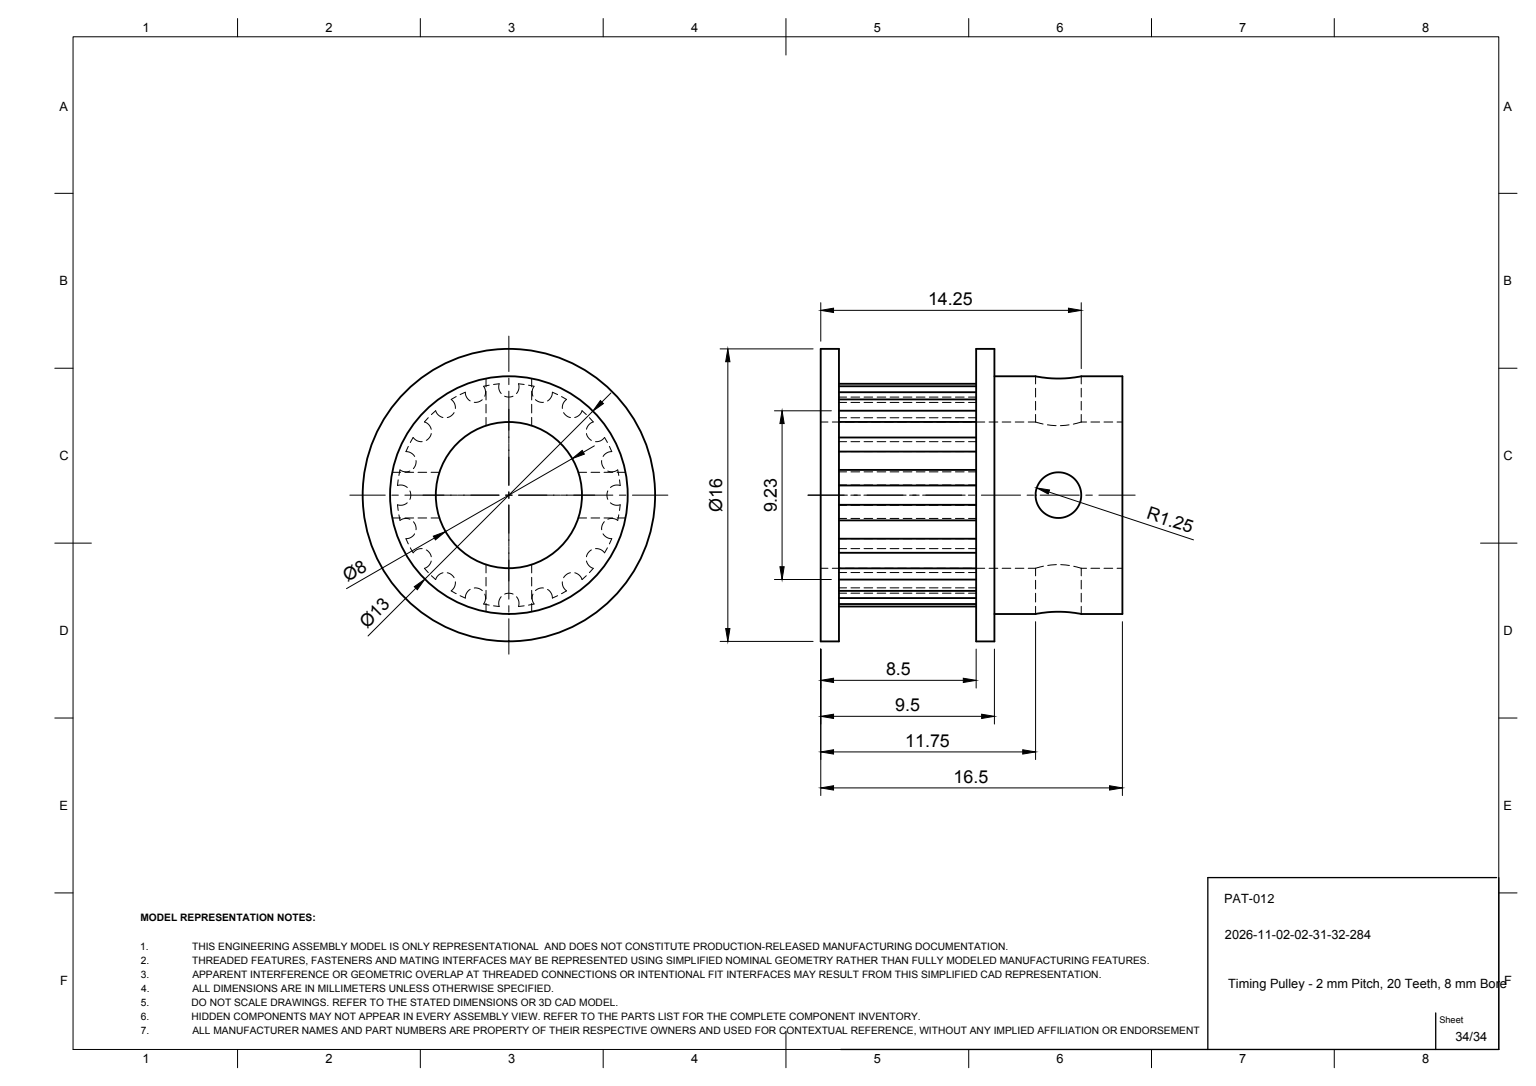
ISO-10303-21;
HEADER;
/* Generated by software containing ST-Developer
 * from STEP Tools, Inc. (www.steptools.com) 
 */

FILE_DESCRIPTION(
/* description */ ('Belt tensioner idler arm'),
/* implementation_level */ '2;1');

FILE_NAME(
/* name */ 'Timing Pulley - 2 mm Pitch, 20 Teeth, 8 mm Bore.step',
/* time_stamp */ '2026-10-28T03:22:15-07:00',
/* author */ (''),
/* organization */ (''),
/* preprocessor_version */ 'ST-DEVELOPER v20.2',
/* originating_system */ 'Autodesk Translation Framework v15.17.0.0',
/* authorisation */ '');

FILE_SCHEMA (('AUTOMOTIVE_DESIGN { 1 0 10303 214 3 1 1 }'));
ENDSEC;

DATA;
#10=MECHANICAL_DESIGN_GEOMETRIC_PRESENTATION_REPRESENTATION('',(#487),#12779);
#357=B_SPLINE_CURVE_WITH_KNOTS('',3,(#12023,#12024,#12025,#12026,#12027,
#12028,#12029,#12030,#12031,#12032),.UNSPECIFIED.,.F.,.F.,(4,2,2,2,4),(0.566550474129931,
0.613761886174531,0.66097329821913,0.708186965196186,0.755400632173242),
 .UNSPECIFIED.);
#358=B_SPLINE_CURVE_WITH_KNOTS('',3,(#12034,#12035,#12036,#12037,#12038,
#12039,#12040,#12041,#12042,#12043,#12044,#12045,#12046,#12047,#12048,#12049,
#12050,#12051),.UNSPECIFIED.,.F.,.F.,(4,2,2,2,2,2,2,2,4),(0.18885015804331,
0.23606157008791,0.283272982132509,0.330486649109565,0.377700316086621,
0.424913983063677,0.472127650040732,0.519339062085332,0.566550474129931),
 .UNSPECIFIED.);
#359=B_SPLINE_CURVE_WITH_KNOTS('',3,(#12052,#12053,#12054,#12055,#12056,
#12057,#12058,#12059,#12060,#12061),.UNSPECIFIED.,.F.,.F.,(4,2,2,2,4),(0.755400632173242,
0.802614299150298,0.849827966127353,0.897039378171953,0.944250790216552),
 .UNSPECIFIED.);
#360=B_SPLINE_CURVE_WITH_KNOTS('',3,(#12065,#12066,#12067,#12068,#12069,
#12070,#12071,#12072,#12073,#12074),.UNSPECIFIED.,.F.,.F.,(4,2,2,2,4),(0.189723673274825,
0.237146208024627,0.28456874277443,0.33200804466204,0.37944734654965),
 .UNSPECIFIED.);
#361=B_SPLINE_CURVE_WITH_KNOTS('',3,(#12076,#12077,#12078,#12079,#12080,
#12081,#12082,#12083,#12084,#12085),.UNSPECIFIED.,.F.,.F.,(4,2,2,2,4),(0.,
0.0474393018876097,0.0948786037752193,0.142301138525022,0.189723673274825),
 .UNSPECIFIED.);
#362=B_SPLINE_CURVE_WITH_KNOTS('',3,(#12087,#12088,#12089,#12090,#12091,
#12092,#12093,#12094,#12095,#12096),.UNSPECIFIED.,.F.,.F.,(4,2,2,2,4),(0.569171019824474,
0.616593554574277,0.66401608932408,0.711455391211689,0.758894693099299),
 .UNSPECIFIED.);
#363=B_SPLINE_CURVE_WITH_KNOTS('',3,(#12097,#12098,#12099,#12100,#12101,
#12102,#12103,#12104,#12105,#12106),.UNSPECIFIED.,.F.,.F.,(4,2,2,2,4),(0.37944734654965,
0.426886648437259,0.474325950324869,0.521748485074671,0.569171019824474),
 .UNSPECIFIED.);
#364=B_SPLINE_CURVE_WITH_KNOTS('',3,(#12110,#12111,#12112,#12113,#12114,
#12115,#12116,#12117,#12118,#12119,#12120,#12121,#12122,#12123,#12124,#12125,
#12126,#12127),.UNSPECIFIED.,.F.,.F.,(4,2,2,2,2,2,2,2,4),(0.,0.0474393018876097,
0.0948786037752194,0.142301138525022,0.189723673274825,0.237146208024628,
0.28456874277443,0.33200804466204,0.37944734654965),.UNSPECIFIED.);
#365=B_SPLINE_CURVE_WITH_KNOTS('',3,(#12128,#12129,#12130,#12131,#12132,
#12133,#12134,#12135,#12136,#12137,#12138,#12139,#12140,#12141,#12142,#12143,
#12144,#12145),.UNSPECIFIED.,.F.,.F.,(4,2,2,2,2,2,2,2,4),(0.37944734654965,
0.426886648437259,0.474325950324869,0.521748485074672,0.569171019824474,
0.616593554574277,0.66401608932408,0.711455391211689,0.758894693099299),
 .UNSPECIFIED.);
#366=B_SPLINE_CURVE_WITH_KNOTS('',3,(#12149,#12150,#12151,#12152,#12153,
#12154,#12155,#12156,#12157,#12158),.UNSPECIFIED.,.F.,.F.,(4,2,2,2,4),(0.566550474129931,
0.613761886174531,0.66097329821913,0.708186965196186,0.755400632173242),
 .UNSPECIFIED.);
#367=B_SPLINE_CURVE_WITH_KNOTS('',3,(#12160,#12161,#12162,#12163,#12164,
#12165,#12166,#12167,#12168,#12169,#12170,#12171,#12172,#12173,#12174,#12175,
#12176,#12177),.UNSPECIFIED.,.F.,.F.,(4,2,2,2,2,2,2,2,4),(0.188850158043311,
0.23606157008791,0.283272982132509,0.330486649109565,0.377700316086621,
0.424913983063677,0.472127650040733,0.519339062085332,0.566550474129931),
 .UNSPECIFIED.);
#368=B_SPLINE_CURVE_WITH_KNOTS('',3,(#12178,#12179,#12180,#12181,#12182,
#12183,#12184,#12185,#12186,#12187),.UNSPECIFIED.,.F.,.F.,(4,2,2,2,4),(0.755400632173242,
0.802614299150298,0.849827966127354,0.897039378171953,0.944250790216552),
 .UNSPECIFIED.);
#369=B_SPLINE_CURVE_WITH_KNOTS('',3,(#12197,#12198,#12199,#12200,#12201,
#12202,#12203,#12204,#12205,#12206,#12207,#12208,#12209,#12210,#12211,#12212,
#12213,#12214),.UNSPECIFIED.,.F.,.F.,(4,2,2,2,2,2,2,2,4),(0.18885015804331,
0.23606157008791,0.283272982132509,0.330486649109565,0.377700316086621,
0.424913983063677,0.472127650040732,0.519339062085332,0.566550474129931),
 .UNSPECIFIED.);
#370=B_SPLINE_CURVE_WITH_KNOTS('',3,(#12216,#12217,#12218,#12219,#12220,
#12221,#12222,#12223,#12224,#12225),.UNSPECIFIED.,.F.,.F.,(4,2,2,2,4),(0.566550474129931,
0.613761886174531,0.66097329821913,0.708186965196186,0.755400632173242),
 .UNSPECIFIED.);
#371=B_SPLINE_CURVE_WITH_KNOTS('',3,(#12226,#12227,#12228,#12229,#12230,
#12231,#12232,#12233,#12234,#12235),.UNSPECIFIED.,.F.,.F.,(4,2,2,2,4),(0.755400632173242,
0.802614299150298,0.849827966127353,0.897039378171953,0.944250790216552),
 .UNSPECIFIED.);
#372=B_SPLINE_CURVE_WITH_KNOTS('',3,(#12238,#12239,#12240,#12241,#12242,
#12243,#12244,#12245,#12246,#12247,#12248,#12249,#12250,#12251,#12252,#12253,
#12254,#12255),.UNSPECIFIED.,.F.,.F.,(4,2,2,2,2,2,2,2,4),(0.188850158043311,
0.23606157008791,0.283272982132509,0.330486649109565,0.377700316086621,
0.424913983063677,0.472127650040733,0.519339062085332,0.566550474129932),
 .UNSPECIFIED.);
#373=B_SPLINE_CURVE_WITH_KNOTS('',3,(#12257,#12258,#12259,#12260,#12261,
#12262,#12263,#12264,#12265,#12266),.UNSPECIFIED.,.F.,.F.,(4,2,2,2,4),(0.566550474129932,
0.613761886174531,0.66097329821913,0.708186965196186,0.755400632173242),
 .UNSPECIFIED.);
#374=B_SPLINE_CURVE_WITH_KNOTS('',3,(#12267,#12268,#12269,#12270,#12271,
#12272,#12273,#12274,#12275,#12276),.UNSPECIFIED.,.F.,.F.,(4,2,2,2,4),(0.755400632173242,
0.802614299150298,0.849827966127354,0.897039378171953,0.944250790216552),
 .UNSPECIFIED.);
#375=B_SPLINE_CURVE_WITH_KNOTS('',3,(#12281,#12282,#12283,#12284,#12285,
#12286,#12287,#12288,#12289,#12290,#12291,#12292,#12293,#12294,#12295,#12296,
#12297,#12298),.UNSPECIFIED.,.F.,.F.,(4,2,2,2,2,2,2,2,4),(0.,0.0474393018876097,
0.0948786037752193,0.142301138525022,0.189723673274825,0.237146208024627,
0.28456874277443,0.33200804466204,0.37944734654965),.UNSPECIFIED.);
#376=B_SPLINE_CURVE_WITH_KNOTS('',3,(#12299,#12300,#12301,#12302,#12303,
#12304,#12305,#12306,#12307,#12308,#12309,#12310,#12311,#12312,#12313,#12314,
#12315,#12316),.UNSPECIFIED.,.F.,.F.,(4,2,2,2,2,2,2,2,4),(0.37944734654965,
0.426886648437259,0.474325950324869,0.521748485074672,0.569171019824474,
0.616593554574277,0.66401608932408,0.711455391211689,0.758894693099299),
 .UNSPECIFIED.);
#377=B_SPLINE_CURVE_WITH_KNOTS('',3,(#12320,#12321,#12322,#12323,#12324,
#12325,#12326,#12327,#12328,#12329,#12330,#12331,#12332,#12333,#12334,#12335,
#12336,#12337),.UNSPECIFIED.,.F.,.F.,(4,2,2,2,2,2,2,2,4),(0.,0.0474393018876097,
0.0948786037752194,0.142301138525022,0.189723673274825,0.237146208024627,
0.28456874277443,0.33200804466204,0.37944734654965),.UNSPECIFIED.);
#378=B_SPLINE_CURVE_WITH_KNOTS('',3,(#12338,#12339,#12340,#12341,#12342,
#12343,#12344,#12345,#12346,#12347,#12348,#12349,#12350,#12351,#12352,#12353,
#12354,#12355),.UNSPECIFIED.,.F.,.F.,(4,2,2,2,2,2,2,2,4),(0.37944734654965,
0.426886648437259,0.474325950324869,0.521748485074672,0.569171019824474,
0.616593554574277,0.66401608932408,0.711455391211689,0.758894693099299),
 .UNSPECIFIED.);
#411=SHAPE_REPRESENTATION_RELATIONSHIP('SRR','None',#12960,#445);
#445=ADVANCED_BREP_SHAPE_REPRESENTATION('',(#526),#12777);
#487=STYLED_ITEM('',(#13198),#526);
#526=MANIFOLD_SOLID_BREP('Body1',#6224);
#651=FACE_BOUND('',#1629,.T.);
#652=FACE_BOUND('',#1630,.T.);
#653=FACE_BOUND('',#1631,.T.);
#654=FACE_BOUND('',#1635,.T.);
#655=FACE_BOUND('',#1636,.T.);
#656=FACE_BOUND('',#1637,.T.);
#657=FACE_BOUND('',#1639,.T.);
#658=FACE_BOUND('',#1641,.T.);
#659=FACE_BOUND('',#1644,.T.);
#660=FACE_BOUND('',#1646,.T.);
#661=FACE_BOUND('',#1649,.T.);
#821=PLANE('',#7265);
#822=PLANE('',#7266);
#823=PLANE('',#7310);
#824=PLANE('',#7311);
#825=PLANE('',#7355);
#1135=FACE_OUTER_BOUND('',#1626,.T.);
#1136=FACE_OUTER_BOUND('',#1627,.T.);
#1137=FACE_OUTER_BOUND('',#1628,.T.);
#1138=FACE_OUTER_BOUND('',#1632,.T.);
#1139=FACE_OUTER_BOUND('',#1633,.T.);
#1140=FACE_OUTER_BOUND('',#1634,.T.);
#1141=FACE_OUTER_BOUND('',#1638,.T.);
#1142=FACE_OUTER_BOUND('',#1640,.T.);
#1143=FACE_OUTER_BOUND('',#1642,.T.);
#1144=FACE_OUTER_BOUND('',#1643,.T.);
#1145=FACE_OUTER_BOUND('',#1645,.T.);
#1146=FACE_OUTER_BOUND('',#1647,.T.);
#1147=FACE_OUTER_BOUND('',#1648,.T.);
#1148=FACE_OUTER_BOUND('',#1650,.T.);
#1149=FACE_OUTER_BOUND('',#1651,.T.);
#1150=FACE_OUTER_BOUND('',#1652,.T.);
#1151=FACE_OUTER_BOUND('',#1653,.T.);
#1152=FACE_OUTER_BOUND('',#1654,.T.);
#1153=FACE_OUTER_BOUND('',#1655,.T.);
#1154=FACE_OUTER_BOUND('',#1656,.T.);
#1155=FACE_OUTER_BOUND('',#1657,.T.);
#1156=FACE_OUTER_BOUND('',#1658,.T.);
#1157=FACE_OUTER_BOUND('',#1659,.T.);
#1158=FACE_OUTER_BOUND('',#1660,.T.);
#1159=FACE_OUTER_BOUND('',#1661,.T.);
#1160=FACE_OUTER_BOUND('',#1662,.T.);
#1161=FACE_OUTER_BOUND('',#1663,.T.);
#1162=FACE_OUTER_BOUND('',#1664,.T.);
#1163=FACE_OUTER_BOUND('',#1665,.T.);
#1164=FACE_OUTER_BOUND('',#1666,.T.);
#1165=FACE_OUTER_BOUND('',#1667,.T.);
#1166=FACE_OUTER_BOUND('',#1668,.T.);
#1167=FACE_OUTER_BOUND('',#1669,.T.);
#1168=FACE_OUTER_BOUND('',#1670,.T.);
#1169=FACE_OUTER_BOUND('',#1671,.T.);
#1170=FACE_OUTER_BOUND('',#1672,.T.);
#1171=FACE_OUTER_BOUND('',#1673,.T.);
#1172=FACE_OUTER_BOUND('',#1674,.T.);
#1173=FACE_OUTER_BOUND('',#1675,.T.);
#1174=FACE_OUTER_BOUND('',#1676,.T.);
#1175=FACE_OUTER_BOUND('',#1677,.T.);
#1176=FACE_OUTER_BOUND('',#1678,.T.);
#1177=FACE_OUTER_BOUND('',#1679,.T.);
#1178=FACE_OUTER_BOUND('',#1680,.T.);
#1179=FACE_OUTER_BOUND('',#1681,.T.);
#1180=FACE_OUTER_BOUND('',#1682,.T.);
#1181=FACE_OUTER_BOUND('',#1683,.T.);
#1182=FACE_OUTER_BOUND('',#1684,.T.);
#1183=FACE_OUTER_BOUND('',#1685,.T.);
#1184=FACE_OUTER_BOUND('',#1686,.T.);
#1185=FACE_OUTER_BOUND('',#1687,.T.);
#1186=FACE_OUTER_BOUND('',#1688,.T.);
#1187=FACE_OUTER_BOUND('',#1689,.T.);
#1626=EDGE_LOOP('',(#5282,#5283,#5284,#5285,#5286,#5287,#5288,#5289,#5290));
#1627=EDGE_LOOP('',(#5291,#5292,#5293,#5294,#5295,#5296,#5297));
#1628=EDGE_LOOP('',(#5298,#5299,#5300,#5301,#5302,#5303,#5304,#5305,#5306));
#1629=EDGE_LOOP('',(#5307,#5308,#5309));
#1630=EDGE_LOOP('',(#5310,#5311,#5312));
#1631=EDGE_LOOP('',(#5313,#5314,#5315));
#1632=EDGE_LOOP('',(#5316,#5317,#5318,#5319,#5320,#5321,#5322));
#1633=EDGE_LOOP('',(#5323,#5324,#5325,#5326,#5327,#5328,#5329));
#1634=EDGE_LOOP('',(#5330,#5331,#5332,#5333,#5334,#5335,#5336,#5337,#5338,
#5339));
#1635=EDGE_LOOP('',(#5340,#5341));
#1636=EDGE_LOOP('',(#5342,#5343));
#1637=EDGE_LOOP('',(#5344,#5345));
#1638=EDGE_LOOP('',(#5346));
#1639=EDGE_LOOP('',(#5347));
#1640=EDGE_LOOP('',(#5348));
#1641=EDGE_LOOP('',(#5349,#5350,#5351,#5352,#5353,#5354,#5355,#5356,#5357,
#5358,#5359,#5360,#5361,#5362,#5363,#5364,#5365,#5366,#5367,#5368,#5369,
#5370,#5371,#5372,#5373,#5374,#5375,#5376,#5377,#5378,#5379,#5380,#5381,
#5382,#5383,#5384,#5385,#5386,#5387,#5388));
#1642=EDGE_LOOP('',(#5389,#5390,#5391,#5392));
#1643=EDGE_LOOP('',(#5393));
#1644=EDGE_LOOP('',(#5394));
#1645=EDGE_LOOP('',(#5395));
#1646=EDGE_LOOP('',(#5396,#5397,#5398,#5399,#5400,#5401,#5402,#5403,#5404,
#5405,#5406,#5407,#5408,#5409,#5410,#5411,#5412,#5413,#5414,#5415,#5416,
#5417,#5418,#5419,#5420,#5421,#5422,#5423,#5424,#5425,#5426,#5427,#5428,
#5429,#5430,#5431,#5432,#5433,#5434,#5435));
#1647=EDGE_LOOP('',(#5436,#5437,#5438,#5439));
#1648=EDGE_LOOP('',(#5440));
#1649=EDGE_LOOP('',(#5441));
#1650=EDGE_LOOP('',(#5442,#5443,#5444,#5445));
#1651=EDGE_LOOP('',(#5446,#5447,#5448,#5449));
#1652=EDGE_LOOP('',(#5450,#5451,#5452,#5453));
#1653=EDGE_LOOP('',(#5454,#5455,#5456,#5457));
#1654=EDGE_LOOP('',(#5458,#5459,#5460,#5461));
#1655=EDGE_LOOP('',(#5462,#5463,#5464,#5465));
#1656=EDGE_LOOP('',(#5466,#5467,#5468,#5469));
#1657=EDGE_LOOP('',(#5470,#5471,#5472,#5473));
#1658=EDGE_LOOP('',(#5474,#5475,#5476,#5477));
#1659=EDGE_LOOP('',(#5478,#5479,#5480,#5481));
#1660=EDGE_LOOP('',(#5482,#5483,#5484,#5485));
#1661=EDGE_LOOP('',(#5486,#5487,#5488,#5489));
#1662=EDGE_LOOP('',(#5490,#5491,#5492,#5493));
#1663=EDGE_LOOP('',(#5494,#5495,#5496,#5497));
#1664=EDGE_LOOP('',(#5498,#5499,#5500,#5501));
#1665=EDGE_LOOP('',(#5502,#5503,#5504,#5505));
#1666=EDGE_LOOP('',(#5506,#5507,#5508,#5509));
#1667=EDGE_LOOP('',(#5510,#5511,#5512,#5513));
#1668=EDGE_LOOP('',(#5514,#5515,#5516,#5517));
#1669=EDGE_LOOP('',(#5518,#5519,#5520,#5521));
#1670=EDGE_LOOP('',(#5522,#5523,#5524,#5525));
#1671=EDGE_LOOP('',(#5526,#5527,#5528,#5529));
#1672=EDGE_LOOP('',(#5530,#5531,#5532,#5533));
#1673=EDGE_LOOP('',(#5534,#5535,#5536,#5537));
#1674=EDGE_LOOP('',(#5538,#5539,#5540,#5541));
#1675=EDGE_LOOP('',(#5542,#5543,#5544,#5545));
#1676=EDGE_LOOP('',(#5546,#5547,#5548,#5549));
#1677=EDGE_LOOP('',(#5550,#5551,#5552,#5553));
#1678=EDGE_LOOP('',(#5554,#5555,#5556,#5557));
#1679=EDGE_LOOP('',(#5558,#5559,#5560,#5561));
#1680=EDGE_LOOP('',(#5562,#5563,#5564,#5565));
#1681=EDGE_LOOP('',(#5566,#5567,#5568,#5569));
#1682=EDGE_LOOP('',(#5570,#5571,#5572,#5573));
#1683=EDGE_LOOP('',(#5574,#5575,#5576,#5577));
#1684=EDGE_LOOP('',(#5578,#5579,#5580,#5581));
#1685=EDGE_LOOP('',(#5582,#5583,#5584,#5585));
#1686=EDGE_LOOP('',(#5586,#5587,#5588,#5589));
#1687=EDGE_LOOP('',(#5590,#5591,#5592,#5593));
#1688=EDGE_LOOP('',(#5594,#5595,#5596,#5597));
#1689=EDGE_LOOP('',(#5598,#5599,#5600,#5601));
#1983=LINE('',#12063,#2332);
#1984=LINE('',#12147,#2333);
#1985=LINE('',#12191,#2334);
#1986=LINE('',#12193,#2335);
#1987=LINE('',#12279,#2336);
#1988=LINE('',#12356,#2337);
#1989=LINE('',#12360,#2338);
#1990=LINE('',#12362,#2339);
#1991=LINE('',#12451,#2340);
#1992=LINE('',#12539,#2341);
#1993=LINE('',#12542,#2342);
#1994=LINE('',#12543,#2343);
#1995=LINE('',#12545,#2344);
#1996=LINE('',#12547,#2345);
#1997=LINE('',#12549,#2346);
#1998=LINE('',#12551,#2347);
#1999=LINE('',#12553,#2348);
#2000=LINE('',#12555,#2349);
#2001=LINE('',#12557,#2350);
#2002=LINE('',#12559,#2351);
#2003=LINE('',#12561,#2352);
#2004=LINE('',#12563,#2353);
#2005=LINE('',#12565,#2354);
#2006=LINE('',#12567,#2355);
#2007=LINE('',#12569,#2356);
#2008=LINE('',#12571,#2357);
#2009=LINE('',#12573,#2358);
#2010=LINE('',#12575,#2359);
#2011=LINE('',#12577,#2360);
#2012=LINE('',#12579,#2361);
#2013=LINE('',#12581,#2362);
#2014=LINE('',#12583,#2363);
#2015=LINE('',#12585,#2364);
#2016=LINE('',#12587,#2365);
#2017=LINE('',#12589,#2366);
#2018=LINE('',#12591,#2367);
#2019=LINE('',#12593,#2368);
#2020=LINE('',#12595,#2369);
#2021=LINE('',#12597,#2370);
#2022=LINE('',#12599,#2371);
#2023=LINE('',#12601,#2372);
#2024=LINE('',#12603,#2373);
#2025=LINE('',#12605,#2374);
#2026=LINE('',#12607,#2375);
#2027=LINE('',#12609,#2376);
#2028=LINE('',#12611,#2377);
#2029=LINE('',#12613,#2378);
#2030=LINE('',#12615,#2379);
#2031=LINE('',#12617,#2380);
#2032=LINE('',#12619,#2381);
#2332=VECTOR('',#9017,0.125);
#2333=VECTOR('',#9020,0.125);
#2334=VECTOR('',#9025,0.65);
#2335=VECTOR('',#9026,0.65);
#2336=VECTOR('',#9031,0.125);
#2337=VECTOR('',#9034,0.125);
#2338=VECTOR('',#9039,0.4);
#2339=VECTOR('',#9040,0.4);
#2340=VECTOR('',#9133,0.8);
#2341=VECTOR('',#9224,0.8);
#2342=VECTOR('',#9229,1.);
#2343=VECTOR('',#9230,1.);
#2344=VECTOR('',#9233,1.);
#2345=VECTOR('',#9236,1.);
#2346=VECTOR('',#9239,1.);
#2347=VECTOR('',#9242,1.);
#2348=VECTOR('',#9245,1.);
#2349=VECTOR('',#9248,1.);
#2350=VECTOR('',#9251,1.);
#2351=VECTOR('',#9254,1.);
#2352=VECTOR('',#9257,1.);
#2353=VECTOR('',#9260,1.);
#2354=VECTOR('',#9263,1.);
#2355=VECTOR('',#9266,1.);
#2356=VECTOR('',#9269,1.);
#2357=VECTOR('',#9272,1.);
#2358=VECTOR('',#9275,1.);
#2359=VECTOR('',#9278,1.);
#2360=VECTOR('',#9281,1.);
#2361=VECTOR('',#9284,1.);
#2362=VECTOR('',#9287,1.);
#2363=VECTOR('',#9290,1.);
#2364=VECTOR('',#9293,1.);
#2365=VECTOR('',#9296,1.);
#2366=VECTOR('',#9299,1.);
#2367=VECTOR('',#9302,1.);
#2368=VECTOR('',#9305,1.);
#2369=VECTOR('',#9308,1.);
#2370=VECTOR('',#9311,1.);
#2371=VECTOR('',#9314,1.);
#2372=VECTOR('',#9317,1.);
#2373=VECTOR('',#9320,1.);
#2374=VECTOR('',#9323,1.);
#2375=VECTOR('',#9326,1.);
#2376=VECTOR('',#9329,1.);
#2377=VECTOR('',#9332,1.);
#2378=VECTOR('',#9335,1.);
#2379=VECTOR('',#9338,1.);
#2380=VECTOR('',#9341,1.);
#2381=VECTOR('',#9344,1.);
#2674=CIRCLE('',#7258,0.65);
#2675=CIRCLE('',#7259,0.65);
#2676=CIRCLE('',#7263,0.4);
#2677=CIRCLE('',#7264,0.4);
#2678=CIRCLE('',#7267,0.8);
#2679=CIRCLE('',#7268,0.0555);
#2680=CIRCLE('',#7269,0.611219772367581);
#2681=CIRCLE('',#7270,0.0555);
#2682=CIRCLE('',#7271,0.611219772367581);
#2683=CIRCLE('',#7272,0.0555);
#2684=CIRCLE('',#7273,0.611219772367581);
#2685=CIRCLE('',#7274,0.0555);
#2686=CIRCLE('',#7275,0.611219772367581);
#2687=CIRCLE('',#7276,0.0555);
#2688=CIRCLE('',#7277,0.611219772367581);
#2689=CIRCLE('',#7278,0.0555);
#2690=CIRCLE('',#7279,0.611219772367581);
#2691=CIRCLE('',#7280,0.0555);
#2692=CIRCLE('',#7281,0.611219772367581);
#2693=CIRCLE('',#7282,0.0555);
#2694=CIRCLE('',#7283,0.611219772367581);
#2695=CIRCLE('',#7284,0.0555);
#2696=CIRCLE('',#7285,0.611219772367581);
#2697=CIRCLE('',#7286,0.0555);
#2698=CIRCLE('',#7287,0.611219772367581);
#2699=CIRCLE('',#7288,0.0555);
#2700=CIRCLE('',#7289,0.611219772367581);
#2701=CIRCLE('',#7290,0.0555);
#2702=CIRCLE('',#7291,0.611219772367581);
#2703=CIRCLE('',#7292,0.0555);
#2704=CIRCLE('',#7293,0.611219772367581);
#2705=CIRCLE('',#7294,0.0555);
#2706=CIRCLE('',#7295,0.611219772367581);
#2707=CIRCLE('',#7296,0.0555);
#2708=CIRCLE('',#7297,0.611219772367581);
#2709=CIRCLE('',#7298,0.0555);
#2710=CIRCLE('',#7299,0.611219772367581);
#2711=CIRCLE('',#7300,0.0555);
#2712=CIRCLE('',#7301,0.611219772367581);
#2713=CIRCLE('',#7302,0.0555);
#2714=CIRCLE('',#7303,0.611219772367581);
#2715=CIRCLE('',#7304,0.0555);
#2716=CIRCLE('',#7305,0.611219772367581);
#2717=CIRCLE('',#7306,0.0555);
#2718=CIRCLE('',#7307,0.611219772367581);
#2719=CIRCLE('',#7309,0.8);
#2720=CIRCLE('',#7312,0.8);
#2721=CIRCLE('',#7313,0.0555);
#2722=CIRCLE('',#7314,0.611219772367581);
#2723=CIRCLE('',#7315,0.0555);
#2724=CIRCLE('',#7316,0.611219772367581);
#2725=CIRCLE('',#7317,0.0555);
#2726=CIRCLE('',#7318,0.611219772367581);
#2727=CIRCLE('',#7319,0.0555);
#2728=CIRCLE('',#7320,0.611219772367581);
#2729=CIRCLE('',#7321,0.0555);
#2730=CIRCLE('',#7322,0.611219772367581);
#2731=CIRCLE('',#7323,0.0555);
#2732=CIRCLE('',#7324,0.611219772367581);
#2733=CIRCLE('',#7325,0.0555);
#2734=CIRCLE('',#7326,0.611219772367581);
#2735=CIRCLE('',#7327,0.0555);
#2736=CIRCLE('',#7328,0.611219772367581);
#2737=CIRCLE('',#7329,0.0555);
#2738=CIRCLE('',#7330,0.611219772367581);
#2739=CIRCLE('',#7331,0.0555);
#2740=CIRCLE('',#7332,0.611219772367581);
#2741=CIRCLE('',#7333,0.0555);
#2742=CIRCLE('',#7334,0.611219772367581);
#2743=CIRCLE('',#7335,0.0555);
#2744=CIRCLE('',#7336,0.611219772367581);
#2745=CIRCLE('',#7337,0.0555);
#2746=CIRCLE('',#7338,0.611219772367581);
#2747=CIRCLE('',#7339,0.0555);
#2748=CIRCLE('',#7340,0.611219772367581);
#2749=CIRCLE('',#7341,0.0555);
#2750=CIRCLE('',#7342,0.611219772367581);
#2751=CIRCLE('',#7343,0.0555);
#2752=CIRCLE('',#7344,0.611219772367581);
#2753=CIRCLE('',#7345,0.0555);
#2754=CIRCLE('',#7346,0.611219772367581);
#2755=CIRCLE('',#7347,0.0555);
#2756=CIRCLE('',#7348,0.611219772367581);
#2757=CIRCLE('',#7349,0.0555);
#2758=CIRCLE('',#7350,0.611219772367581);
#2759=CIRCLE('',#7351,0.0555);
#2760=CIRCLE('',#7352,0.611219772367581);
#2761=CIRCLE('',#7354,0.8);
#3169=VERTEX_POINT('',#12021);
#3170=VERTEX_POINT('',#12022);
#3171=VERTEX_POINT('',#12033);
#3172=VERTEX_POINT('',#12062);
#3173=VERTEX_POINT('',#12064);
#3174=VERTEX_POINT('',#12075);
#3175=VERTEX_POINT('',#12086);
#3176=VERTEX_POINT('',#12108);
#3177=VERTEX_POINT('',#12109);
#3178=VERTEX_POINT('',#12146);
#3179=VERTEX_POINT('',#12148);
#3180=VERTEX_POINT('',#12159);
#3181=VERTEX_POINT('',#12189);
#3182=VERTEX_POINT('',#12192);
#3183=VERTEX_POINT('',#12195);
#3184=VERTEX_POINT('',#12196);
#3185=VERTEX_POINT('',#12215);
#3186=VERTEX_POINT('',#12236);
#3187=VERTEX_POINT('',#12237);
#3188=VERTEX_POINT('',#12256);
#3189=VERTEX_POINT('',#12278);
#3190=VERTEX_POINT('',#12280);
#3191=VERTEX_POINT('',#12318);
#3192=VERTEX_POINT('',#12319);
#3193=VERTEX_POINT('',#12358);
#3194=VERTEX_POINT('',#12361);
#3195=VERTEX_POINT('',#12366);
#3196=VERTEX_POINT('',#12368);
#3197=VERTEX_POINT('',#12369);
#3198=VERTEX_POINT('',#12371);
#3199=VERTEX_POINT('',#12373);
#3200=VERTEX_POINT('',#12375);
#3201=VERTEX_POINT('',#12377);
#3202=VERTEX_POINT('',#12379);
#3203=VERTEX_POINT('',#12381);
#3204=VERTEX_POINT('',#12383);
#3205=VERTEX_POINT('',#12385);
#3206=VERTEX_POINT('',#12387);
#3207=VERTEX_POINT('',#12389);
#3208=VERTEX_POINT('',#12391);
#3209=VERTEX_POINT('',#12393);
#3210=VERTEX_POINT('',#12395);
#3211=VERTEX_POINT('',#12397);
#3212=VERTEX_POINT('',#12399);
#3213=VERTEX_POINT('',#12401);
#3214=VERTEX_POINT('',#12403);
#3215=VERTEX_POINT('',#12405);
#3216=VERTEX_POINT('',#12407);
#3217=VERTEX_POINT('',#12409);
#3218=VERTEX_POINT('',#12411);
#3219=VERTEX_POINT('',#12413);
#3220=VERTEX_POINT('',#12415);
#3221=VERTEX_POINT('',#12417);
#3222=VERTEX_POINT('',#12419);
#3223=VERTEX_POINT('',#12421);
#3224=VERTEX_POINT('',#12423);
#3225=VERTEX_POINT('',#12425);
#3226=VERTEX_POINT('',#12427);
#3227=VERTEX_POINT('',#12429);
#3228=VERTEX_POINT('',#12431);
#3229=VERTEX_POINT('',#12433);
#3230=VERTEX_POINT('',#12435);
#3231=VERTEX_POINT('',#12437);
#3232=VERTEX_POINT('',#12439);
#3233=VERTEX_POINT('',#12441);
#3234=VERTEX_POINT('',#12443);
#3235=VERTEX_POINT('',#12445);
#3236=VERTEX_POINT('',#12449);
#3237=VERTEX_POINT('',#12454);
#3238=VERTEX_POINT('',#12456);
#3239=VERTEX_POINT('',#12457);
#3240=VERTEX_POINT('',#12459);
#3241=VERTEX_POINT('',#12461);
#3242=VERTEX_POINT('',#12463);
#3243=VERTEX_POINT('',#12465);
#3244=VERTEX_POINT('',#12467);
#3245=VERTEX_POINT('',#12469);
#3246=VERTEX_POINT('',#12471);
#3247=VERTEX_POINT('',#12473);
#3248=VERTEX_POINT('',#12475);
#3249=VERTEX_POINT('',#12477);
#3250=VERTEX_POINT('',#12479);
#3251=VERTEX_POINT('',#12481);
#3252=VERTEX_POINT('',#12483);
#3253=VERTEX_POINT('',#12485);
#3254=VERTEX_POINT('',#12487);
#3255=VERTEX_POINT('',#12489);
#3256=VERTEX_POINT('',#12491);
#3257=VERTEX_POINT('',#12493);
#3258=VERTEX_POINT('',#12495);
#3259=VERTEX_POINT('',#12497);
#3260=VERTEX_POINT('',#12499);
#3261=VERTEX_POINT('',#12501);
#3262=VERTEX_POINT('',#12503);
#3263=VERTEX_POINT('',#12505);
#3264=VERTEX_POINT('',#12507);
#3265=VERTEX_POINT('',#12509);
#3266=VERTEX_POINT('',#12511);
#3267=VERTEX_POINT('',#12513);
#3268=VERTEX_POINT('',#12515);
#3269=VERTEX_POINT('',#12517);
#3270=VERTEX_POINT('',#12519);
#3271=VERTEX_POINT('',#12521);
#3272=VERTEX_POINT('',#12523);
#3273=VERTEX_POINT('',#12525);
#3274=VERTEX_POINT('',#12527);
#3275=VERTEX_POINT('',#12529);
#3276=VERTEX_POINT('',#12531);
#3277=VERTEX_POINT('',#12533);
#3278=VERTEX_POINT('',#12537);
#3896=EDGE_CURVE('',#3169,#3170,#357,.T.);
#3897=EDGE_CURVE('',#3171,#3169,#358,.T.);
#3898=EDGE_CURVE('',#3170,#3171,#359,.T.);
#3899=EDGE_CURVE('',#3170,#3172,#1983,.T.);
#3900=EDGE_CURVE('',#3173,#3172,#360,.T.);
#3901=EDGE_CURVE('',#3174,#3173,#361,.T.);
#3902=EDGE_CURVE('',#3175,#3174,#362,.T.);
#3903=EDGE_CURVE('',#3172,#3175,#363,.T.);
#3904=EDGE_CURVE('',#3176,#3177,#364,.T.);
#3905=EDGE_CURVE('',#3177,#3176,#365,.T.);
#3906=EDGE_CURVE('',#3177,#3178,#1984,.T.);
#3907=EDGE_CURVE('',#3179,#3178,#366,.T.);
#3908=EDGE_CURVE('',#3180,#3179,#367,.T.);
#3909=EDGE_CURVE('',#3178,#3180,#368,.T.);
#3910=EDGE_CURVE('',#3181,#3181,#2674,.T.);
#3911=EDGE_CURVE('',#3181,#3171,#1985,.T.);
#3912=EDGE_CURVE('',#3169,#3182,#1986,.T.);
#3913=EDGE_CURVE('',#3182,#3182,#2675,.T.);
#3914=EDGE_CURVE('',#3183,#3184,#369,.T.);
#3915=EDGE_CURVE('',#3184,#3185,#370,.T.);
#3916=EDGE_CURVE('',#3185,#3183,#371,.T.);
#3917=EDGE_CURVE('',#3186,#3187,#372,.T.);
#3918=EDGE_CURVE('',#3187,#3188,#373,.T.);
#3919=EDGE_CURVE('',#3188,#3186,#374,.T.);
#3920=EDGE_CURVE('',#3185,#3189,#1987,.T.);
#3921=EDGE_CURVE('',#3190,#3189,#375,.T.);
#3922=EDGE_CURVE('',#3189,#3190,#376,.T.);
#3923=EDGE_CURVE('',#3191,#3192,#377,.T.);
#3924=EDGE_CURVE('',#3192,#3191,#378,.T.);
#3925=EDGE_CURVE('',#3192,#3188,#1988,.T.);
#3926=EDGE_CURVE('',#3193,#3193,#2676,.T.);
#3927=EDGE_CURVE('',#3193,#3173,#1989,.T.);
#3928=EDGE_CURVE('',#3175,#3194,#1990,.T.);
#3929=EDGE_CURVE('',#3194,#3194,#2677,.T.);
#3930=EDGE_CURVE('',#3195,#3195,#2678,.T.);
#3931=EDGE_CURVE('',#3196,#3197,#2679,.T.);
#3932=EDGE_CURVE('',#3198,#3197,#2680,.T.);
#3933=EDGE_CURVE('',#3198,#3199,#2681,.T.);
#3934=EDGE_CURVE('',#3200,#3199,#2682,.T.);
#3935=EDGE_CURVE('',#3200,#3201,#2683,.T.);
#3936=EDGE_CURVE('',#3202,#3201,#2684,.T.);
#3937=EDGE_CURVE('',#3202,#3203,#2685,.T.);
#3938=EDGE_CURVE('',#3204,#3203,#2686,.T.);
#3939=EDGE_CURVE('',#3204,#3205,#2687,.T.);
#3940=EDGE_CURVE('',#3206,#3205,#2688,.T.);
#3941=EDGE_CURVE('',#3206,#3207,#2689,.T.);
#3942=EDGE_CURVE('',#3208,#3207,#2690,.T.);
#3943=EDGE_CURVE('',#3208,#3209,#2691,.T.);
#3944=EDGE_CURVE('',#3210,#3209,#2692,.T.);
#3945=EDGE_CURVE('',#3210,#3211,#2693,.T.);
#3946=EDGE_CURVE('',#3212,#3211,#2694,.T.);
#3947=EDGE_CURVE('',#3212,#3213,#2695,.T.);
#3948=EDGE_CURVE('',#3214,#3213,#2696,.T.);
#3949=EDGE_CURVE('',#3214,#3215,#2697,.T.);
#3950=EDGE_CURVE('',#3216,#3215,#2698,.T.);
#3951=EDGE_CURVE('',#3216,#3217,#2699,.T.);
#3952=EDGE_CURVE('',#3218,#3217,#2700,.T.);
#3953=EDGE_CURVE('',#3218,#3219,#2701,.T.);
#3954=EDGE_CURVE('',#3220,#3219,#2702,.T.);
#3955=EDGE_CURVE('',#3220,#3221,#2703,.T.);
#3956=EDGE_CURVE('',#3222,#3221,#2704,.T.);
#3957=EDGE_CURVE('',#3222,#3223,#2705,.T.);
#3958=EDGE_CURVE('',#3224,#3223,#2706,.T.);
#3959=EDGE_CURVE('',#3224,#3225,#2707,.T.);
#3960=EDGE_CURVE('',#3226,#3225,#2708,.T.);
#3961=EDGE_CURVE('',#3226,#3227,#2709,.T.);
#3962=EDGE_CURVE('',#3228,#3227,#2710,.T.);
#3963=EDGE_CURVE('',#3228,#3229,#2711,.T.);
#3964=EDGE_CURVE('',#3230,#3229,#2712,.T.);
#3965=EDGE_CURVE('',#3230,#3231,#2713,.T.);
#3966=EDGE_CURVE('',#3232,#3231,#2714,.T.);
#3967=EDGE_CURVE('',#3232,#3233,#2715,.T.);
#3968=EDGE_CURVE('',#3234,#3233,#2716,.T.);
#3969=EDGE_CURVE('',#3234,#3235,#2717,.T.);
#3970=EDGE_CURVE('',#3196,#3235,#2718,.T.);
#3971=EDGE_CURVE('',#3236,#3236,#2719,.T.);
#3972=EDGE_CURVE('',#3236,#3195,#1991,.T.);
#3973=EDGE_CURVE('',#3237,#3237,#2720,.T.);
#3974=EDGE_CURVE('',#3238,#3239,#2721,.T.);
#3975=EDGE_CURVE('',#3239,#3240,#2722,.T.);
#3976=EDGE_CURVE('',#3240,#3241,#2723,.T.);
#3977=EDGE_CURVE('',#3241,#3242,#2724,.T.);
#3978=EDGE_CURVE('',#3242,#3243,#2725,.T.);
#3979=EDGE_CURVE('',#3243,#3244,#2726,.T.);
#3980=EDGE_CURVE('',#3244,#3245,#2727,.T.);
#3981=EDGE_CURVE('',#3245,#3246,#2728,.T.);
#3982=EDGE_CURVE('',#3246,#3247,#2729,.T.);
#3983=EDGE_CURVE('',#3247,#3248,#2730,.T.);
#3984=EDGE_CURVE('',#3248,#3249,#2731,.T.);
#3985=EDGE_CURVE('',#3249,#3250,#2732,.T.);
#3986=EDGE_CURVE('',#3250,#3251,#2733,.T.);
#3987=EDGE_CURVE('',#3251,#3252,#2734,.T.);
#3988=EDGE_CURVE('',#3252,#3253,#2735,.T.);
#3989=EDGE_CURVE('',#3253,#3254,#2736,.T.);
#3990=EDGE_CURVE('',#3254,#3255,#2737,.T.);
#3991=EDGE_CURVE('',#3255,#3256,#2738,.T.);
#3992=EDGE_CURVE('',#3256,#3257,#2739,.T.);
#3993=EDGE_CURVE('',#3257,#3258,#2740,.T.);
#3994=EDGE_CURVE('',#3258,#3259,#2741,.T.);
#3995=EDGE_CURVE('',#3259,#3260,#2742,.T.);
#3996=EDGE_CURVE('',#3260,#3261,#2743,.T.);
#3997=EDGE_CURVE('',#3261,#3262,#2744,.T.);
#3998=EDGE_CURVE('',#3262,#3263,#2745,.T.);
#3999=EDGE_CURVE('',#3263,#3264,#2746,.T.);
#4000=EDGE_CURVE('',#3264,#3265,#2747,.T.);
#4001=EDGE_CURVE('',#3265,#3266,#2748,.T.);
#4002=EDGE_CURVE('',#3266,#3267,#2749,.T.);
#4003=EDGE_CURVE('',#3267,#3268,#2750,.T.);
#4004=EDGE_CURVE('',#3268,#3269,#2751,.T.);
#4005=EDGE_CURVE('',#3269,#3270,#2752,.T.);
#4006=EDGE_CURVE('',#3270,#3271,#2753,.T.);
#4007=EDGE_CURVE('',#3271,#3272,#2754,.T.);
#4008=EDGE_CURVE('',#3272,#3273,#2755,.T.);
#4009=EDGE_CURVE('',#3273,#3274,#2756,.T.);
#4010=EDGE_CURVE('',#3274,#3275,#2757,.T.);
#4011=EDGE_CURVE('',#3275,#3276,#2758,.T.);
#4012=EDGE_CURVE('',#3276,#3277,#2759,.T.);
#4013=EDGE_CURVE('',#3277,#3238,#2760,.T.);
#4014=EDGE_CURVE('',#3278,#3278,#2761,.T.);
#4015=EDGE_CURVE('',#3278,#3237,#1992,.T.);
#4016=EDGE_CURVE('',#3239,#3196,#1993,.T.);
#4017=EDGE_CURVE('',#3197,#3238,#1994,.T.);
#4018=EDGE_CURVE('',#3277,#3198,#1995,.T.);
#4019=EDGE_CURVE('',#3199,#3276,#1996,.T.);
#4020=EDGE_CURVE('',#3275,#3200,#1997,.T.);
#4021=EDGE_CURVE('',#3201,#3274,#1998,.T.);
#4022=EDGE_CURVE('',#3273,#3202,#1999,.T.);
#4023=EDGE_CURVE('',#3203,#3272,#2000,.T.);
#4024=EDGE_CURVE('',#3271,#3204,#2001,.T.);
#4025=EDGE_CURVE('',#3205,#3270,#2002,.T.);
#4026=EDGE_CURVE('',#3269,#3206,#2003,.T.);
#4027=EDGE_CURVE('',#3207,#3268,#2004,.T.);
#4028=EDGE_CURVE('',#3267,#3208,#2005,.T.);
#4029=EDGE_CURVE('',#3209,#3266,#2006,.T.);
#4030=EDGE_CURVE('',#3265,#3210,#2007,.T.);
#4031=EDGE_CURVE('',#3211,#3264,#2008,.T.);
#4032=EDGE_CURVE('',#3263,#3212,#2009,.T.);
#4033=EDGE_CURVE('',#3213,#3262,#2010,.T.);
#4034=EDGE_CURVE('',#3261,#3214,#2011,.T.);
#4035=EDGE_CURVE('',#3215,#3260,#2012,.T.);
#4036=EDGE_CURVE('',#3259,#3216,#2013,.T.);
#4037=EDGE_CURVE('',#3217,#3258,#2014,.T.);
#4038=EDGE_CURVE('',#3257,#3218,#2015,.T.);
#4039=EDGE_CURVE('',#3219,#3256,#2016,.T.);
#4040=EDGE_CURVE('',#3255,#3220,#2017,.T.);
#4041=EDGE_CURVE('',#3221,#3254,#2018,.T.);
#4042=EDGE_CURVE('',#3253,#3222,#2019,.T.);
#4043=EDGE_CURVE('',#3223,#3252,#2020,.T.);
#4044=EDGE_CURVE('',#3251,#3224,#2021,.T.);
#4045=EDGE_CURVE('',#3225,#3250,#2022,.T.);
#4046=EDGE_CURVE('',#3249,#3226,#2023,.T.);
#4047=EDGE_CURVE('',#3227,#3248,#2024,.T.);
#4048=EDGE_CURVE('',#3247,#3228,#2025,.T.);
#4049=EDGE_CURVE('',#3229,#3246,#2026,.T.);
#4050=EDGE_CURVE('',#3245,#3230,#2027,.T.);
#4051=EDGE_CURVE('',#3231,#3244,#2028,.T.);
#4052=EDGE_CURVE('',#3243,#3232,#2029,.T.);
#4053=EDGE_CURVE('',#3233,#3242,#2030,.T.);
#4054=EDGE_CURVE('',#3235,#3240,#2031,.T.);
#4055=EDGE_CURVE('',#3241,#3234,#2032,.T.);
#5282=ORIENTED_EDGE('',*,*,#3896,.F.);
#5283=ORIENTED_EDGE('',*,*,#3897,.F.);
#5284=ORIENTED_EDGE('',*,*,#3898,.F.);
#5285=ORIENTED_EDGE('',*,*,#3899,.T.);
#5286=ORIENTED_EDGE('',*,*,#3900,.F.);
#5287=ORIENTED_EDGE('',*,*,#3901,.F.);
#5288=ORIENTED_EDGE('',*,*,#3902,.F.);
#5289=ORIENTED_EDGE('',*,*,#3903,.F.);
#5290=ORIENTED_EDGE('',*,*,#3899,.F.);
#5291=ORIENTED_EDGE('',*,*,#3904,.F.);
#5292=ORIENTED_EDGE('',*,*,#3905,.F.);
#5293=ORIENTED_EDGE('',*,*,#3906,.T.);
#5294=ORIENTED_EDGE('',*,*,#3907,.F.);
#5295=ORIENTED_EDGE('',*,*,#3908,.F.);
#5296=ORIENTED_EDGE('',*,*,#3909,.F.);
#5297=ORIENTED_EDGE('',*,*,#3906,.F.);
#5298=ORIENTED_EDGE('',*,*,#3910,.F.);
#5299=ORIENTED_EDGE('',*,*,#3911,.T.);
#5300=ORIENTED_EDGE('',*,*,#3897,.T.);
#5301=ORIENTED_EDGE('',*,*,#3912,.T.);
#5302=ORIENTED_EDGE('',*,*,#3913,.F.);
#5303=ORIENTED_EDGE('',*,*,#3912,.F.);
#5304=ORIENTED_EDGE('',*,*,#3896,.T.);
#5305=ORIENTED_EDGE('',*,*,#3898,.T.);
#5306=ORIENTED_EDGE('',*,*,#3911,.F.);
#5307=ORIENTED_EDGE('',*,*,#3908,.T.);
#5308=ORIENTED_EDGE('',*,*,#3907,.T.);
#5309=ORIENTED_EDGE('',*,*,#3909,.T.);
#5310=ORIENTED_EDGE('',*,*,#3914,.T.);
#5311=ORIENTED_EDGE('',*,*,#3915,.T.);
#5312=ORIENTED_EDGE('',*,*,#3916,.T.);
#5313=ORIENTED_EDGE('',*,*,#3917,.T.);
#5314=ORIENTED_EDGE('',*,*,#3918,.T.);
#5315=ORIENTED_EDGE('',*,*,#3919,.T.);
#5316=ORIENTED_EDGE('',*,*,#3915,.F.);
#5317=ORIENTED_EDGE('',*,*,#3914,.F.);
#5318=ORIENTED_EDGE('',*,*,#3916,.F.);
#5319=ORIENTED_EDGE('',*,*,#3920,.T.);
#5320=ORIENTED_EDGE('',*,*,#3921,.F.);
#5321=ORIENTED_EDGE('',*,*,#3922,.F.);
#5322=ORIENTED_EDGE('',*,*,#3920,.F.);
#5323=ORIENTED_EDGE('',*,*,#3923,.F.);
#5324=ORIENTED_EDGE('',*,*,#3924,.F.);
#5325=ORIENTED_EDGE('',*,*,#3925,.T.);
#5326=ORIENTED_EDGE('',*,*,#3918,.F.);
#5327=ORIENTED_EDGE('',*,*,#3917,.F.);
#5328=ORIENTED_EDGE('',*,*,#3919,.F.);
#5329=ORIENTED_EDGE('',*,*,#3925,.F.);
#5330=ORIENTED_EDGE('',*,*,#3926,.F.);
#5331=ORIENTED_EDGE('',*,*,#3927,.T.);
#5332=ORIENTED_EDGE('',*,*,#3900,.T.);
#5333=ORIENTED_EDGE('',*,*,#3903,.T.);
#5334=ORIENTED_EDGE('',*,*,#3928,.T.);
#5335=ORIENTED_EDGE('',*,*,#3929,.F.);
#5336=ORIENTED_EDGE('',*,*,#3928,.F.);
#5337=ORIENTED_EDGE('',*,*,#3902,.T.);
#5338=ORIENTED_EDGE('',*,*,#3901,.T.);
#5339=ORIENTED_EDGE('',*,*,#3927,.F.);
#5340=ORIENTED_EDGE('',*,*,#3904,.T.);
#5341=ORIENTED_EDGE('',*,*,#3905,.T.);
#5342=ORIENTED_EDGE('',*,*,#3923,.T.);
#5343=ORIENTED_EDGE('',*,*,#3924,.T.);
#5344=ORIENTED_EDGE('',*,*,#3921,.T.);
#5345=ORIENTED_EDGE('',*,*,#3922,.T.);
#5346=ORIENTED_EDGE('',*,*,#3910,.T.);
#5347=ORIENTED_EDGE('',*,*,#3926,.T.);
#5348=ORIENTED_EDGE('',*,*,#3930,.T.);
#5349=ORIENTED_EDGE('',*,*,#3931,.T.);
#5350=ORIENTED_EDGE('',*,*,#3932,.F.);
#5351=ORIENTED_EDGE('',*,*,#3933,.T.);
#5352=ORIENTED_EDGE('',*,*,#3934,.F.);
#5353=ORIENTED_EDGE('',*,*,#3935,.T.);
#5354=ORIENTED_EDGE('',*,*,#3936,.F.);
#5355=ORIENTED_EDGE('',*,*,#3937,.T.);
#5356=ORIENTED_EDGE('',*,*,#3938,.F.);
#5357=ORIENTED_EDGE('',*,*,#3939,.T.);
#5358=ORIENTED_EDGE('',*,*,#3940,.F.);
#5359=ORIENTED_EDGE('',*,*,#3941,.T.);
#5360=ORIENTED_EDGE('',*,*,#3942,.F.);
#5361=ORIENTED_EDGE('',*,*,#3943,.T.);
#5362=ORIENTED_EDGE('',*,*,#3944,.F.);
#5363=ORIENTED_EDGE('',*,*,#3945,.T.);
#5364=ORIENTED_EDGE('',*,*,#3946,.F.);
#5365=ORIENTED_EDGE('',*,*,#3947,.T.);
#5366=ORIENTED_EDGE('',*,*,#3948,.F.);
#5367=ORIENTED_EDGE('',*,*,#3949,.T.);
#5368=ORIENTED_EDGE('',*,*,#3950,.F.);
#5369=ORIENTED_EDGE('',*,*,#3951,.T.);
#5370=ORIENTED_EDGE('',*,*,#3952,.F.);
#5371=ORIENTED_EDGE('',*,*,#3953,.T.);
#5372=ORIENTED_EDGE('',*,*,#3954,.F.);
#5373=ORIENTED_EDGE('',*,*,#3955,.T.);
#5374=ORIENTED_EDGE('',*,*,#3956,.F.);
#5375=ORIENTED_EDGE('',*,*,#3957,.T.);
#5376=ORIENTED_EDGE('',*,*,#3958,.F.);
#5377=ORIENTED_EDGE('',*,*,#3959,.T.);
#5378=ORIENTED_EDGE('',*,*,#3960,.F.);
#5379=ORIENTED_EDGE('',*,*,#3961,.T.);
#5380=ORIENTED_EDGE('',*,*,#3962,.F.);
#5381=ORIENTED_EDGE('',*,*,#3963,.T.);
#5382=ORIENTED_EDGE('',*,*,#3964,.F.);
#5383=ORIENTED_EDGE('',*,*,#3965,.T.);
#5384=ORIENTED_EDGE('',*,*,#3966,.F.);
#5385=ORIENTED_EDGE('',*,*,#3967,.T.);
#5386=ORIENTED_EDGE('',*,*,#3968,.F.);
#5387=ORIENTED_EDGE('',*,*,#3969,.T.);
#5388=ORIENTED_EDGE('',*,*,#3970,.F.);
#5389=ORIENTED_EDGE('',*,*,#3971,.F.);
#5390=ORIENTED_EDGE('',*,*,#3972,.T.);
#5391=ORIENTED_EDGE('',*,*,#3930,.F.);
#5392=ORIENTED_EDGE('',*,*,#3972,.F.);
#5393=ORIENTED_EDGE('',*,*,#3971,.T.);
#5394=ORIENTED_EDGE('',*,*,#3913,.T.);
#5395=ORIENTED_EDGE('',*,*,#3973,.F.);
#5396=ORIENTED_EDGE('',*,*,#3974,.T.);
#5397=ORIENTED_EDGE('',*,*,#3975,.T.);
#5398=ORIENTED_EDGE('',*,*,#3976,.T.);
#5399=ORIENTED_EDGE('',*,*,#3977,.T.);
#5400=ORIENTED_EDGE('',*,*,#3978,.T.);
#5401=ORIENTED_EDGE('',*,*,#3979,.T.);
#5402=ORIENTED_EDGE('',*,*,#3980,.T.);
#5403=ORIENTED_EDGE('',*,*,#3981,.T.);
#5404=ORIENTED_EDGE('',*,*,#3982,.T.);
#5405=ORIENTED_EDGE('',*,*,#3983,.T.);
#5406=ORIENTED_EDGE('',*,*,#3984,.T.);
#5407=ORIENTED_EDGE('',*,*,#3985,.T.);
#5408=ORIENTED_EDGE('',*,*,#3986,.T.);
#5409=ORIENTED_EDGE('',*,*,#3987,.T.);
#5410=ORIENTED_EDGE('',*,*,#3988,.T.);
#5411=ORIENTED_EDGE('',*,*,#3989,.T.);
#5412=ORIENTED_EDGE('',*,*,#3990,.T.);
#5413=ORIENTED_EDGE('',*,*,#3991,.T.);
#5414=ORIENTED_EDGE('',*,*,#3992,.T.);
#5415=ORIENTED_EDGE('',*,*,#3993,.T.);
#5416=ORIENTED_EDGE('',*,*,#3994,.T.);
#5417=ORIENTED_EDGE('',*,*,#3995,.T.);
#5418=ORIENTED_EDGE('',*,*,#3996,.T.);
#5419=ORIENTED_EDGE('',*,*,#3997,.T.);
#5420=ORIENTED_EDGE('',*,*,#3998,.T.);
#5421=ORIENTED_EDGE('',*,*,#3999,.T.);
#5422=ORIENTED_EDGE('',*,*,#4000,.T.);
#5423=ORIENTED_EDGE('',*,*,#4001,.T.);
#5424=ORIENTED_EDGE('',*,*,#4002,.T.);
#5425=ORIENTED_EDGE('',*,*,#4003,.T.);
#5426=ORIENTED_EDGE('',*,*,#4004,.T.);
#5427=ORIENTED_EDGE('',*,*,#4005,.T.);
#5428=ORIENTED_EDGE('',*,*,#4006,.T.);
#5429=ORIENTED_EDGE('',*,*,#4007,.T.);
#5430=ORIENTED_EDGE('',*,*,#4008,.T.);
#5431=ORIENTED_EDGE('',*,*,#4009,.T.);
#5432=ORIENTED_EDGE('',*,*,#4010,.T.);
#5433=ORIENTED_EDGE('',*,*,#4011,.T.);
#5434=ORIENTED_EDGE('',*,*,#4012,.T.);
#5435=ORIENTED_EDGE('',*,*,#4013,.T.);
#5436=ORIENTED_EDGE('',*,*,#4014,.F.);
#5437=ORIENTED_EDGE('',*,*,#4015,.T.);
#5438=ORIENTED_EDGE('',*,*,#3973,.T.);
#5439=ORIENTED_EDGE('',*,*,#4015,.F.);
#5440=ORIENTED_EDGE('',*,*,#4014,.T.);
#5441=ORIENTED_EDGE('',*,*,#3929,.T.);
#5442=ORIENTED_EDGE('',*,*,#4016,.F.);
#5443=ORIENTED_EDGE('',*,*,#3974,.F.);
#5444=ORIENTED_EDGE('',*,*,#4017,.F.);
#5445=ORIENTED_EDGE('',*,*,#3931,.F.);
#5446=ORIENTED_EDGE('',*,*,#4017,.T.);
#5447=ORIENTED_EDGE('',*,*,#4013,.F.);
#5448=ORIENTED_EDGE('',*,*,#4018,.T.);
#5449=ORIENTED_EDGE('',*,*,#3932,.T.);
#5450=ORIENTED_EDGE('',*,*,#4018,.F.);
#5451=ORIENTED_EDGE('',*,*,#4012,.F.);
#5452=ORIENTED_EDGE('',*,*,#4019,.F.);
#5453=ORIENTED_EDGE('',*,*,#3933,.F.);
#5454=ORIENTED_EDGE('',*,*,#4019,.T.);
#5455=ORIENTED_EDGE('',*,*,#4011,.F.);
#5456=ORIENTED_EDGE('',*,*,#4020,.T.);
#5457=ORIENTED_EDGE('',*,*,#3934,.T.);
#5458=ORIENTED_EDGE('',*,*,#4020,.F.);
#5459=ORIENTED_EDGE('',*,*,#4010,.F.);
#5460=ORIENTED_EDGE('',*,*,#4021,.F.);
#5461=ORIENTED_EDGE('',*,*,#3935,.F.);
#5462=ORIENTED_EDGE('',*,*,#4021,.T.);
#5463=ORIENTED_EDGE('',*,*,#4009,.F.);
#5464=ORIENTED_EDGE('',*,*,#4022,.T.);
#5465=ORIENTED_EDGE('',*,*,#3936,.T.);
#5466=ORIENTED_EDGE('',*,*,#4022,.F.);
#5467=ORIENTED_EDGE('',*,*,#4008,.F.);
#5468=ORIENTED_EDGE('',*,*,#4023,.F.);
#5469=ORIENTED_EDGE('',*,*,#3937,.F.);
#5470=ORIENTED_EDGE('',*,*,#4023,.T.);
#5471=ORIENTED_EDGE('',*,*,#4007,.F.);
#5472=ORIENTED_EDGE('',*,*,#4024,.T.);
#5473=ORIENTED_EDGE('',*,*,#3938,.T.);
#5474=ORIENTED_EDGE('',*,*,#4024,.F.);
#5475=ORIENTED_EDGE('',*,*,#4006,.F.);
#5476=ORIENTED_EDGE('',*,*,#4025,.F.);
#5477=ORIENTED_EDGE('',*,*,#3939,.F.);
#5478=ORIENTED_EDGE('',*,*,#4025,.T.);
#5479=ORIENTED_EDGE('',*,*,#4005,.F.);
#5480=ORIENTED_EDGE('',*,*,#4026,.T.);
#5481=ORIENTED_EDGE('',*,*,#3940,.T.);
#5482=ORIENTED_EDGE('',*,*,#4026,.F.);
#5483=ORIENTED_EDGE('',*,*,#4004,.F.);
#5484=ORIENTED_EDGE('',*,*,#4027,.F.);
#5485=ORIENTED_EDGE('',*,*,#3941,.F.);
#5486=ORIENTED_EDGE('',*,*,#4027,.T.);
#5487=ORIENTED_EDGE('',*,*,#4003,.F.);
#5488=ORIENTED_EDGE('',*,*,#4028,.T.);
#5489=ORIENTED_EDGE('',*,*,#3942,.T.);
#5490=ORIENTED_EDGE('',*,*,#4028,.F.);
#5491=ORIENTED_EDGE('',*,*,#4002,.F.);
#5492=ORIENTED_EDGE('',*,*,#4029,.F.);
#5493=ORIENTED_EDGE('',*,*,#3943,.F.);
#5494=ORIENTED_EDGE('',*,*,#4029,.T.);
#5495=ORIENTED_EDGE('',*,*,#4001,.F.);
#5496=ORIENTED_EDGE('',*,*,#4030,.T.);
#5497=ORIENTED_EDGE('',*,*,#3944,.T.);
#5498=ORIENTED_EDGE('',*,*,#4030,.F.);
#5499=ORIENTED_EDGE('',*,*,#4000,.F.);
#5500=ORIENTED_EDGE('',*,*,#4031,.F.);
#5501=ORIENTED_EDGE('',*,*,#3945,.F.);
#5502=ORIENTED_EDGE('',*,*,#4031,.T.);
#5503=ORIENTED_EDGE('',*,*,#3999,.F.);
#5504=ORIENTED_EDGE('',*,*,#4032,.T.);
#5505=ORIENTED_EDGE('',*,*,#3946,.T.);
#5506=ORIENTED_EDGE('',*,*,#4032,.F.);
#5507=ORIENTED_EDGE('',*,*,#3998,.F.);
#5508=ORIENTED_EDGE('',*,*,#4033,.F.);
#5509=ORIENTED_EDGE('',*,*,#3947,.F.);
#5510=ORIENTED_EDGE('',*,*,#4033,.T.);
#5511=ORIENTED_EDGE('',*,*,#3997,.F.);
#5512=ORIENTED_EDGE('',*,*,#4034,.T.);
#5513=ORIENTED_EDGE('',*,*,#3948,.T.);
#5514=ORIENTED_EDGE('',*,*,#4034,.F.);
#5515=ORIENTED_EDGE('',*,*,#3996,.F.);
#5516=ORIENTED_EDGE('',*,*,#4035,.F.);
#5517=ORIENTED_EDGE('',*,*,#3949,.F.);
#5518=ORIENTED_EDGE('',*,*,#4035,.T.);
#5519=ORIENTED_EDGE('',*,*,#3995,.F.);
#5520=ORIENTED_EDGE('',*,*,#4036,.T.);
#5521=ORIENTED_EDGE('',*,*,#3950,.T.);
#5522=ORIENTED_EDGE('',*,*,#4036,.F.);
#5523=ORIENTED_EDGE('',*,*,#3994,.F.);
#5524=ORIENTED_EDGE('',*,*,#4037,.F.);
#5525=ORIENTED_EDGE('',*,*,#3951,.F.);
#5526=ORIENTED_EDGE('',*,*,#4037,.T.);
#5527=ORIENTED_EDGE('',*,*,#3993,.F.);
#5528=ORIENTED_EDGE('',*,*,#4038,.T.);
#5529=ORIENTED_EDGE('',*,*,#3952,.T.);
#5530=ORIENTED_EDGE('',*,*,#4038,.F.);
#5531=ORIENTED_EDGE('',*,*,#3992,.F.);
#5532=ORIENTED_EDGE('',*,*,#4039,.F.);
#5533=ORIENTED_EDGE('',*,*,#3953,.F.);
#5534=ORIENTED_EDGE('',*,*,#4039,.T.);
#5535=ORIENTED_EDGE('',*,*,#3991,.F.);
#5536=ORIENTED_EDGE('',*,*,#4040,.T.);
#5537=ORIENTED_EDGE('',*,*,#3954,.T.);
#5538=ORIENTED_EDGE('',*,*,#4040,.F.);
#5539=ORIENTED_EDGE('',*,*,#3990,.F.);
#5540=ORIENTED_EDGE('',*,*,#4041,.F.);
#5541=ORIENTED_EDGE('',*,*,#3955,.F.);
#5542=ORIENTED_EDGE('',*,*,#4041,.T.);
#5543=ORIENTED_EDGE('',*,*,#3989,.F.);
#5544=ORIENTED_EDGE('',*,*,#4042,.T.);
#5545=ORIENTED_EDGE('',*,*,#3956,.T.);
#5546=ORIENTED_EDGE('',*,*,#4042,.F.);
#5547=ORIENTED_EDGE('',*,*,#3988,.F.);
#5548=ORIENTED_EDGE('',*,*,#4043,.F.);
#5549=ORIENTED_EDGE('',*,*,#3957,.F.);
#5550=ORIENTED_EDGE('',*,*,#4043,.T.);
#5551=ORIENTED_EDGE('',*,*,#3987,.F.);
#5552=ORIENTED_EDGE('',*,*,#4044,.T.);
#5553=ORIENTED_EDGE('',*,*,#3958,.T.);
#5554=ORIENTED_EDGE('',*,*,#4044,.F.);
#5555=ORIENTED_EDGE('',*,*,#3986,.F.);
#5556=ORIENTED_EDGE('',*,*,#4045,.F.);
#5557=ORIENTED_EDGE('',*,*,#3959,.F.);
#5558=ORIENTED_EDGE('',*,*,#4045,.T.);
#5559=ORIENTED_EDGE('',*,*,#3985,.F.);
#5560=ORIENTED_EDGE('',*,*,#4046,.T.);
#5561=ORIENTED_EDGE('',*,*,#3960,.T.);
#5562=ORIENTED_EDGE('',*,*,#4046,.F.);
#5563=ORIENTED_EDGE('',*,*,#3984,.F.);
#5564=ORIENTED_EDGE('',*,*,#4047,.F.);
#5565=ORIENTED_EDGE('',*,*,#3961,.F.);
#5566=ORIENTED_EDGE('',*,*,#4047,.T.);
#5567=ORIENTED_EDGE('',*,*,#3983,.F.);
#5568=ORIENTED_EDGE('',*,*,#4048,.T.);
#5569=ORIENTED_EDGE('',*,*,#3962,.T.);
#5570=ORIENTED_EDGE('',*,*,#4048,.F.);
#5571=ORIENTED_EDGE('',*,*,#3982,.F.);
#5572=ORIENTED_EDGE('',*,*,#4049,.F.);
#5573=ORIENTED_EDGE('',*,*,#3963,.F.);
#5574=ORIENTED_EDGE('',*,*,#4049,.T.);
#5575=ORIENTED_EDGE('',*,*,#3981,.F.);
#5576=ORIENTED_EDGE('',*,*,#4050,.T.);
#5577=ORIENTED_EDGE('',*,*,#3964,.T.);
#5578=ORIENTED_EDGE('',*,*,#4050,.F.);
#5579=ORIENTED_EDGE('',*,*,#3980,.F.);
#5580=ORIENTED_EDGE('',*,*,#4051,.F.);
#5581=ORIENTED_EDGE('',*,*,#3965,.F.);
#5582=ORIENTED_EDGE('',*,*,#4051,.T.);
#5583=ORIENTED_EDGE('',*,*,#3979,.F.);
#5584=ORIENTED_EDGE('',*,*,#4052,.T.);
#5585=ORIENTED_EDGE('',*,*,#3966,.T.);
#5586=ORIENTED_EDGE('',*,*,#4053,.F.);
#5587=ORIENTED_EDGE('',*,*,#3967,.F.);
#5588=ORIENTED_EDGE('',*,*,#4052,.F.);
#5589=ORIENTED_EDGE('',*,*,#3978,.F.);
#5590=ORIENTED_EDGE('',*,*,#4016,.T.);
#5591=ORIENTED_EDGE('',*,*,#3970,.T.);
#5592=ORIENTED_EDGE('',*,*,#4054,.T.);
#5593=ORIENTED_EDGE('',*,*,#3975,.F.);
#5594=ORIENTED_EDGE('',*,*,#4055,.F.);
#5595=ORIENTED_EDGE('',*,*,#3976,.F.);
#5596=ORIENTED_EDGE('',*,*,#4054,.F.);
#5597=ORIENTED_EDGE('',*,*,#3969,.F.);
#5598=ORIENTED_EDGE('',*,*,#4053,.T.);
#5599=ORIENTED_EDGE('',*,*,#3977,.F.);
#5600=ORIENTED_EDGE('',*,*,#4055,.T.);
#5601=ORIENTED_EDGE('',*,*,#3968,.T.);
#5764=CYLINDRICAL_SURFACE('',#7255,0.125);
#5765=CYLINDRICAL_SURFACE('',#7256,0.125);
#5766=CYLINDRICAL_SURFACE('',#7257,0.65);
#5767=CYLINDRICAL_SURFACE('',#7260,0.125);
#5768=CYLINDRICAL_SURFACE('',#7261,0.125);
#5769=CYLINDRICAL_SURFACE('',#7262,0.4);
#5770=CYLINDRICAL_SURFACE('',#7308,0.8);
#5771=CYLINDRICAL_SURFACE('',#7353,0.8);
#5772=CYLINDRICAL_SURFACE('',#7356,0.0555);
#5773=CYLINDRICAL_SURFACE('',#7357,0.611219772367581);
#5774=CYLINDRICAL_SURFACE('',#7358,0.0555);
#5775=CYLINDRICAL_SURFACE('',#7359,0.611219772367581);
#5776=CYLINDRICAL_SURFACE('',#7360,0.0555);
#5777=CYLINDRICAL_SURFACE('',#7361,0.611219772367581);
#5778=CYLINDRICAL_SURFACE('',#7362,0.0555);
#5779=CYLINDRICAL_SURFACE('',#7363,0.611219772367581);
#5780=CYLINDRICAL_SURFACE('',#7364,0.0555);
#5781=CYLINDRICAL_SURFACE('',#7365,0.611219772367581);
#5782=CYLINDRICAL_SURFACE('',#7366,0.0555);
#5783=CYLINDRICAL_SURFACE('',#7367,0.611219772367581);
#5784=CYLINDRICAL_SURFACE('',#7368,0.0555);
#5785=CYLINDRICAL_SURFACE('',#7369,0.611219772367581);
#5786=CYLINDRICAL_SURFACE('',#7370,0.0555);
#5787=CYLINDRICAL_SURFACE('',#7371,0.611219772367581);
#5788=CYLINDRICAL_SURFACE('',#7372,0.0555);
#5789=CYLINDRICAL_SURFACE('',#7373,0.611219772367581);
#5790=CYLINDRICAL_SURFACE('',#7374,0.0555);
#5791=CYLINDRICAL_SURFACE('',#7375,0.611219772367581);
#5792=CYLINDRICAL_SURFACE('',#7376,0.0555);
#5793=CYLINDRICAL_SURFACE('',#7377,0.611219772367581);
#5794=CYLINDRICAL_SURFACE('',#7378,0.0555);
#5795=CYLINDRICAL_SURFACE('',#7379,0.611219772367581);
#5796=CYLINDRICAL_SURFACE('',#7380,0.0555);
#5797=CYLINDRICAL_SURFACE('',#7381,0.611219772367581);
#5798=CYLINDRICAL_SURFACE('',#7382,0.0555);
#5799=CYLINDRICAL_SURFACE('',#7383,0.611219772367581);
#5800=CYLINDRICAL_SURFACE('',#7384,0.0555);
#5801=CYLINDRICAL_SURFACE('',#7385,0.611219772367581);
#5802=CYLINDRICAL_SURFACE('',#7386,0.0555);
#5803=CYLINDRICAL_SURFACE('',#7387,0.611219772367581);
#5804=CYLINDRICAL_SURFACE('',#7388,0.0555);
#5805=CYLINDRICAL_SURFACE('',#7389,0.611219772367581);
#5806=CYLINDRICAL_SURFACE('',#7390,0.0555);
#5807=CYLINDRICAL_SURFACE('',#7391,0.611219772367581);
#5808=CYLINDRICAL_SURFACE('',#7392,0.0555);
#5809=CYLINDRICAL_SURFACE('',#7393,0.611219772367581);
#5810=CYLINDRICAL_SURFACE('',#7394,0.0555);
#5811=CYLINDRICAL_SURFACE('',#7395,0.611219772367581);
#6112=ADVANCED_FACE('',(#1135),#5764,.F.);
#6113=ADVANCED_FACE('',(#1136),#5765,.F.);
#6114=ADVANCED_FACE('',(#1137,#651,#652,#653),#5766,.T.);
#6115=ADVANCED_FACE('',(#1138),#5767,.F.);
#6116=ADVANCED_FACE('',(#1139),#5768,.F.);
#6117=ADVANCED_FACE('',(#1140,#654,#655,#656),#5769,.F.);
#6118=ADVANCED_FACE('',(#1141,#657),#821,.F.);
#6119=ADVANCED_FACE('',(#1142,#658),#822,.T.);
#6120=ADVANCED_FACE('',(#1143),#5770,.T.);
#6121=ADVANCED_FACE('',(#1144,#659),#823,.F.);
#6122=ADVANCED_FACE('',(#1145,#660),#824,.F.);
#6123=ADVANCED_FACE('',(#1146),#5771,.T.);
#6124=ADVANCED_FACE('',(#1147,#661),#825,.T.);
#6125=ADVANCED_FACE('',(#1148),#5772,.F.);
#6126=ADVANCED_FACE('',(#1149),#5773,.T.);
#6127=ADVANCED_FACE('',(#1150),#5774,.F.);
#6128=ADVANCED_FACE('',(#1151),#5775,.T.);
#6129=ADVANCED_FACE('',(#1152),#5776,.F.);
#6130=ADVANCED_FACE('',(#1153),#5777,.T.);
#6131=ADVANCED_FACE('',(#1154),#5778,.F.);
#6132=ADVANCED_FACE('',(#1155),#5779,.T.);
#6133=ADVANCED_FACE('',(#1156),#5780,.F.);
#6134=ADVANCED_FACE('',(#1157),#5781,.T.);
#6135=ADVANCED_FACE('',(#1158),#5782,.F.);
#6136=ADVANCED_FACE('',(#1159),#5783,.T.);
#6137=ADVANCED_FACE('',(#1160),#5784,.F.);
#6138=ADVANCED_FACE('',(#1161),#5785,.T.);
#6139=ADVANCED_FACE('',(#1162),#5786,.F.);
#6140=ADVANCED_FACE('',(#1163),#5787,.T.);
#6141=ADVANCED_FACE('',(#1164),#5788,.F.);
#6142=ADVANCED_FACE('',(#1165),#5789,.T.);
#6143=ADVANCED_FACE('',(#1166),#5790,.F.);
#6144=ADVANCED_FACE('',(#1167),#5791,.T.);
#6145=ADVANCED_FACE('',(#1168),#5792,.F.);
#6146=ADVANCED_FACE('',(#1169),#5793,.T.);
#6147=ADVANCED_FACE('',(#1170),#5794,.F.);
#6148=ADVANCED_FACE('',(#1171),#5795,.T.);
#6149=ADVANCED_FACE('',(#1172),#5796,.F.);
#6150=ADVANCED_FACE('',(#1173),#5797,.T.);
#6151=ADVANCED_FACE('',(#1174),#5798,.F.);
#6152=ADVANCED_FACE('',(#1175),#5799,.T.);
#6153=ADVANCED_FACE('',(#1176),#5800,.F.);
#6154=ADVANCED_FACE('',(#1177),#5801,.T.);
#6155=ADVANCED_FACE('',(#1178),#5802,.F.);
#6156=ADVANCED_FACE('',(#1179),#5803,.T.);
#6157=ADVANCED_FACE('',(#1180),#5804,.F.);
#6158=ADVANCED_FACE('',(#1181),#5805,.T.);
#6159=ADVANCED_FACE('',(#1182),#5806,.F.);
#6160=ADVANCED_FACE('',(#1183),#5807,.T.);
#6161=ADVANCED_FACE('',(#1184),#5808,.F.);
#6162=ADVANCED_FACE('',(#1185),#5809,.T.);
#6163=ADVANCED_FACE('',(#1186),#5810,.F.);
#6164=ADVANCED_FACE('',(#1187),#5811,.T.);
#6224=CLOSED_SHELL('',(#6112,#6113,#6114,#6115,#6116,#6117,#6118,#6119,
#6120,#6121,#6122,#6123,#6124,#6125,#6126,#6127,#6128,#6129,#6130,#6131,
#6132,#6133,#6134,#6135,#6136,#6137,#6138,#6139,#6140,#6141,#6142,#6143,
#6144,#6145,#6146,#6147,#6148,#6149,#6150,#6151,#6152,#6153,#6154,#6155,
#6156,#6157,#6158,#6159,#6160,#6161,#6162,#6163,#6164));
#7254=AXIS2_PLACEMENT_3D('',#12019,#9013,#9014);
#7255=AXIS2_PLACEMENT_3D('',#12020,#9015,#9016);
#7256=AXIS2_PLACEMENT_3D('',#12107,#9018,#9019);
#7257=AXIS2_PLACEMENT_3D('',#12188,#9021,#9022);
#7258=AXIS2_PLACEMENT_3D('',#12190,#9023,#9024);
#7259=AXIS2_PLACEMENT_3D('',#12194,#9027,#9028);
#7260=AXIS2_PLACEMENT_3D('',#12277,#9029,#9030);
#7261=AXIS2_PLACEMENT_3D('',#12317,#9032,#9033);
#7262=AXIS2_PLACEMENT_3D('',#12357,#9035,#9036);
#7263=AXIS2_PLACEMENT_3D('',#12359,#9037,#9038);
#7264=AXIS2_PLACEMENT_3D('',#12363,#9041,#9042);
#7265=AXIS2_PLACEMENT_3D('',#12364,#9043,#9044);
#7266=AXIS2_PLACEMENT_3D('',#12365,#9045,#9046);
#7267=AXIS2_PLACEMENT_3D('',#12367,#9047,#9048);
#7268=AXIS2_PLACEMENT_3D('',#12370,#9049,#9050);
#7269=AXIS2_PLACEMENT_3D('',#12372,#9051,#9052);
#7270=AXIS2_PLACEMENT_3D('',#12374,#9053,#9054);
#7271=AXIS2_PLACEMENT_3D('',#12376,#9055,#9056);
#7272=AXIS2_PLACEMENT_3D('',#12378,#9057,#9058);
#7273=AXIS2_PLACEMENT_3D('',#12380,#9059,#9060);
#7274=AXIS2_PLACEMENT_3D('',#12382,#9061,#9062);
#7275=AXIS2_PLACEMENT_3D('',#12384,#9063,#9064);
#7276=AXIS2_PLACEMENT_3D('',#12386,#9065,#9066);
#7277=AXIS2_PLACEMENT_3D('',#12388,#9067,#9068);
#7278=AXIS2_PLACEMENT_3D('',#12390,#9069,#9070);
#7279=AXIS2_PLACEMENT_3D('',#12392,#9071,#9072);
#7280=AXIS2_PLACEMENT_3D('',#12394,#9073,#9074);
#7281=AXIS2_PLACEMENT_3D('',#12396,#9075,#9076);
#7282=AXIS2_PLACEMENT_3D('',#12398,#9077,#9078);
#7283=AXIS2_PLACEMENT_3D('',#12400,#9079,#9080);
#7284=AXIS2_PLACEMENT_3D('',#12402,#9081,#9082);
#7285=AXIS2_PLACEMENT_3D('',#12404,#9083,#9084);
#7286=AXIS2_PLACEMENT_3D('',#12406,#9085,#9086);
#7287=AXIS2_PLACEMENT_3D('',#12408,#9087,#9088);
#7288=AXIS2_PLACEMENT_3D('',#12410,#9089,#9090);
#7289=AXIS2_PLACEMENT_3D('',#12412,#9091,#9092);
#7290=AXIS2_PLACEMENT_3D('',#12414,#9093,#9094);
#7291=AXIS2_PLACEMENT_3D('',#12416,#9095,#9096);
#7292=AXIS2_PLACEMENT_3D('',#12418,#9097,#9098);
#7293=AXIS2_PLACEMENT_3D('',#12420,#9099,#9100);
#7294=AXIS2_PLACEMENT_3D('',#12422,#9101,#9102);
#7295=AXIS2_PLACEMENT_3D('',#12424,#9103,#9104);
#7296=AXIS2_PLACEMENT_3D('',#12426,#9105,#9106);
#7297=AXIS2_PLACEMENT_3D('',#12428,#9107,#9108);
#7298=AXIS2_PLACEMENT_3D('',#12430,#9109,#9110);
#7299=AXIS2_PLACEMENT_3D('',#12432,#9111,#9112);
#7300=AXIS2_PLACEMENT_3D('',#12434,#9113,#9114);
#7301=AXIS2_PLACEMENT_3D('',#12436,#9115,#9116);
#7302=AXIS2_PLACEMENT_3D('',#12438,#9117,#9118);
#7303=AXIS2_PLACEMENT_3D('',#12440,#9119,#9120);
#7304=AXIS2_PLACEMENT_3D('',#12442,#9121,#9122);
#7305=AXIS2_PLACEMENT_3D('',#12444,#9123,#9124);
#7306=AXIS2_PLACEMENT_3D('',#12446,#9125,#9126);
#7307=AXIS2_PLACEMENT_3D('',#12447,#9127,#9128);
#7308=AXIS2_PLACEMENT_3D('',#12448,#9129,#9130);
#7309=AXIS2_PLACEMENT_3D('',#12450,#9131,#9132);
#7310=AXIS2_PLACEMENT_3D('',#12452,#9134,#9135);
#7311=AXIS2_PLACEMENT_3D('',#12453,#9136,#9137);
#7312=AXIS2_PLACEMENT_3D('',#12455,#9138,#9139);
#7313=AXIS2_PLACEMENT_3D('',#12458,#9140,#9141);
#7314=AXIS2_PLACEMENT_3D('',#12460,#9142,#9143);
#7315=AXIS2_PLACEMENT_3D('',#12462,#9144,#9145);
#7316=AXIS2_PLACEMENT_3D('',#12464,#9146,#9147);
#7317=AXIS2_PLACEMENT_3D('',#12466,#9148,#9149);
#7318=AXIS2_PLACEMENT_3D('',#12468,#9150,#9151);
#7319=AXIS2_PLACEMENT_3D('',#12470,#9152,#9153);
#7320=AXIS2_PLACEMENT_3D('',#12472,#9154,#9155);
#7321=AXIS2_PLACEMENT_3D('',#12474,#9156,#9157);
#7322=AXIS2_PLACEMENT_3D('',#12476,#9158,#9159);
#7323=AXIS2_PLACEMENT_3D('',#12478,#9160,#9161);
#7324=AXIS2_PLACEMENT_3D('',#12480,#9162,#9163);
#7325=AXIS2_PLACEMENT_3D('',#12482,#9164,#9165);
#7326=AXIS2_PLACEMENT_3D('',#12484,#9166,#9167);
#7327=AXIS2_PLACEMENT_3D('',#12486,#9168,#9169);
#7328=AXIS2_PLACEMENT_3D('',#12488,#9170,#9171);
#7329=AXIS2_PLACEMENT_3D('',#12490,#9172,#9173);
#7330=AXIS2_PLACEMENT_3D('',#12492,#9174,#9175);
#7331=AXIS2_PLACEMENT_3D('',#12494,#9176,#9177);
#7332=AXIS2_PLACEMENT_3D('',#12496,#9178,#9179);
#7333=AXIS2_PLACEMENT_3D('',#12498,#9180,#9181);
#7334=AXIS2_PLACEMENT_3D('',#12500,#9182,#9183);
#7335=AXIS2_PLACEMENT_3D('',#12502,#9184,#9185);
#7336=AXIS2_PLACEMENT_3D('',#12504,#9186,#9187);
#7337=AXIS2_PLACEMENT_3D('',#12506,#9188,#9189);
#7338=AXIS2_PLACEMENT_3D('',#12508,#9190,#9191);
#7339=AXIS2_PLACEMENT_3D('',#12510,#9192,#9193);
#7340=AXIS2_PLACEMENT_3D('',#12512,#9194,#9195);
#7341=AXIS2_PLACEMENT_3D('',#12514,#9196,#9197);
#7342=AXIS2_PLACEMENT_3D('',#12516,#9198,#9199);
#7343=AXIS2_PLACEMENT_3D('',#12518,#9200,#9201);
#7344=AXIS2_PLACEMENT_3D('',#12520,#9202,#9203);
#7345=AXIS2_PLACEMENT_3D('',#12522,#9204,#9205);
#7346=AXIS2_PLACEMENT_3D('',#12524,#9206,#9207);
#7347=AXIS2_PLACEMENT_3D('',#12526,#9208,#9209);
#7348=AXIS2_PLACEMENT_3D('',#12528,#9210,#9211);
#7349=AXIS2_PLACEMENT_3D('',#12530,#9212,#9213);
#7350=AXIS2_PLACEMENT_3D('',#12532,#9214,#9215);
#7351=AXIS2_PLACEMENT_3D('',#12534,#9216,#9217);
#7352=AXIS2_PLACEMENT_3D('',#12535,#9218,#9219);
#7353=AXIS2_PLACEMENT_3D('',#12536,#9220,#9221);
#7354=AXIS2_PLACEMENT_3D('',#12538,#9222,#9223);
#7355=AXIS2_PLACEMENT_3D('',#12540,#9225,#9226);
#7356=AXIS2_PLACEMENT_3D('',#12541,#9227,#9228);
#7357=AXIS2_PLACEMENT_3D('',#12544,#9231,#9232);
#7358=AXIS2_PLACEMENT_3D('',#12546,#9234,#9235);
#7359=AXIS2_PLACEMENT_3D('',#12548,#9237,#9238);
#7360=AXIS2_PLACEMENT_3D('',#12550,#9240,#9241);
#7361=AXIS2_PLACEMENT_3D('',#12552,#9243,#9244);
#7362=AXIS2_PLACEMENT_3D('',#12554,#9246,#9247);
#7363=AXIS2_PLACEMENT_3D('',#12556,#9249,#9250);
#7364=AXIS2_PLACEMENT_3D('',#12558,#9252,#9253);
#7365=AXIS2_PLACEMENT_3D('',#12560,#9255,#9256);
#7366=AXIS2_PLACEMENT_3D('',#12562,#9258,#9259);
#7367=AXIS2_PLACEMENT_3D('',#12564,#9261,#9262);
#7368=AXIS2_PLACEMENT_3D('',#12566,#9264,#9265);
#7369=AXIS2_PLACEMENT_3D('',#12568,#9267,#9268);
#7370=AXIS2_PLACEMENT_3D('',#12570,#9270,#9271);
#7371=AXIS2_PLACEMENT_3D('',#12572,#9273,#9274);
#7372=AXIS2_PLACEMENT_3D('',#12574,#9276,#9277);
#7373=AXIS2_PLACEMENT_3D('',#12576,#9279,#9280);
#7374=AXIS2_PLACEMENT_3D('',#12578,#9282,#9283);
#7375=AXIS2_PLACEMENT_3D('',#12580,#9285,#9286);
#7376=AXIS2_PLACEMENT_3D('',#12582,#9288,#9289);
#7377=AXIS2_PLACEMENT_3D('',#12584,#9291,#9292);
#7378=AXIS2_PLACEMENT_3D('',#12586,#9294,#9295);
#7379=AXIS2_PLACEMENT_3D('',#12588,#9297,#9298);
#7380=AXIS2_PLACEMENT_3D('',#12590,#9300,#9301);
#7381=AXIS2_PLACEMENT_3D('',#12592,#9303,#9304);
#7382=AXIS2_PLACEMENT_3D('',#12594,#9306,#9307);
#7383=AXIS2_PLACEMENT_3D('',#12596,#9309,#9310);
#7384=AXIS2_PLACEMENT_3D('',#12598,#9312,#9313);
#7385=AXIS2_PLACEMENT_3D('',#12600,#9315,#9316);
#7386=AXIS2_PLACEMENT_3D('',#12602,#9318,#9319);
#7387=AXIS2_PLACEMENT_3D('',#12604,#9321,#9322);
#7388=AXIS2_PLACEMENT_3D('',#12606,#9324,#9325);
#7389=AXIS2_PLACEMENT_3D('',#12608,#9327,#9328);
#7390=AXIS2_PLACEMENT_3D('',#12610,#9330,#9331);
#7391=AXIS2_PLACEMENT_3D('',#12612,#9333,#9334);
#7392=AXIS2_PLACEMENT_3D('',#12614,#9336,#9337);
#7393=AXIS2_PLACEMENT_3D('',#12616,#9339,#9340);
#7394=AXIS2_PLACEMENT_3D('',#12618,#9342,#9343);
#7395=AXIS2_PLACEMENT_3D('',#12620,#9345,#9346);
#9013=DIRECTION('axis',(0.,0.,1.));
#9014=DIRECTION('refdir',(1.,0.,0.));
#9015=DIRECTION('center_axis',(1.,0.,6.12323399573677E-17));
#9016=DIRECTION('ref_axis',(6.12323399573677E-17,0.,-1.));
#9017=DIRECTION('',(1.,0.,6.12323399573677E-17));
#9018=DIRECTION('center_axis',(1.,0.,6.12323399573677E-17));
#9019=DIRECTION('ref_axis',(6.12323399573677E-17,0.,-1.));
#9020=DIRECTION('',(1.,0.,6.12323399573677E-17));
#9021=DIRECTION('center_axis',(0.,-1.,0.));
#9022=DIRECTION('ref_axis',(1.,0.,0.));
#9023=DIRECTION('center_axis',(0.,-1.,0.));
#9024=DIRECTION('ref_axis',(1.,0.,0.));
#9025=DIRECTION('',(0.,1.,0.));
#9026=DIRECTION('',(0.,1.,0.));
#9027=DIRECTION('center_axis',(0.,1.,0.));
#9028=DIRECTION('ref_axis',(1.,0.,0.));
#9029=DIRECTION('center_axis',(0.,0.,1.));
#9030=DIRECTION('ref_axis',(1.,0.,0.));
#9031=DIRECTION('',(0.,0.,1.));
#9032=DIRECTION('center_axis',(0.,0.,1.));
#9033=DIRECTION('ref_axis',(1.,0.,0.));
#9034=DIRECTION('',(0.,0.,1.));
#9035=DIRECTION('center_axis',(0.,1.,0.));
#9036=DIRECTION('ref_axis',(1.,0.,0.));
#9037=DIRECTION('center_axis',(0.,1.,0.));
#9038=DIRECTION('ref_axis',(1.,0.,0.));
#9039=DIRECTION('',(0.,1.,0.));
#9040=DIRECTION('',(0.,1.,0.));
#9041=DIRECTION('center_axis',(0.,-1.,0.));
#9042=DIRECTION('ref_axis',(1.,0.,0.));
#9043=DIRECTION('center_axis',(0.,1.,0.));
#9044=DIRECTION('ref_axis',(1.,0.,0.));
#9045=DIRECTION('center_axis',(0.,1.,0.));
#9046=DIRECTION('ref_axis',(1.,0.,0.));
#9047=DIRECTION('center_axis',(0.,1.,0.));
#9048=DIRECTION('ref_axis',(1.,0.,0.));
#9049=DIRECTION('center_axis',(0.,1.,0.));
#9050=DIRECTION('ref_axis',(0.951056516295154,0.,0.309016994374948));
#9051=DIRECTION('center_axis',(0.,1.,0.));
#9052=DIRECTION('ref_axis',(1.,0.,0.));
#9053=DIRECTION('center_axis',(0.,1.,0.));
#9054=DIRECTION('ref_axis',(0.809016994374947,0.,0.587785252292473));
#9055=DIRECTION('center_axis',(0.,1.,0.));
#9056=DIRECTION('ref_axis',(1.,0.,0.));
#9057=DIRECTION('center_axis',(0.,1.,0.));
#9058=DIRECTION('ref_axis',(0.587785252292473,0.,0.809016994374948));
#9059=DIRECTION('center_axis',(0.,1.,0.));
#9060=DIRECTION('ref_axis',(1.,0.,0.));
#9061=DIRECTION('center_axis',(0.,1.,0.));
#9062=DIRECTION('ref_axis',(0.309016994374947,0.,0.951056516295154));
#9063=DIRECTION('center_axis',(0.,1.,0.));
#9064=DIRECTION('ref_axis',(1.,0.,0.));
#9065=DIRECTION('center_axis',(0.,1.,0.));
#9066=DIRECTION('ref_axis',(-1.83697019872103E-16,0.,1.));
#9067=DIRECTION('center_axis',(0.,1.,0.));
#9068=DIRECTION('ref_axis',(1.,0.,0.));
#9069=DIRECTION('center_axis',(0.,1.,0.));
#9070=DIRECTION('ref_axis',(-0.309016994374948,0.,0.951056516295154));
#9071=DIRECTION('center_axis',(0.,1.,0.));
#9072=DIRECTION('ref_axis',(1.,0.,0.));
#9073=DIRECTION('center_axis',(0.,1.,0.));
#9074=DIRECTION('ref_axis',(-0.587785252292473,0.,0.809016994374947));
#9075=DIRECTION('center_axis',(0.,1.,0.));
#9076=DIRECTION('ref_axis',(1.,0.,0.));
#9077=DIRECTION('center_axis',(0.,1.,0.));
#9078=DIRECTION('ref_axis',(-0.809016994374947,0.,0.587785252292473));
#9079=DIRECTION('center_axis',(0.,1.,0.));
#9080=DIRECTION('ref_axis',(1.,0.,0.));
#9081=DIRECTION('center_axis',(0.,1.,0.));
#9082=DIRECTION('ref_axis',(-0.951056516295154,0.,0.309016994374947));
#9083=DIRECTION('center_axis',(0.,1.,0.));
#9084=DIRECTION('ref_axis',(1.,0.,0.));
#9085=DIRECTION('center_axis',(0.,1.,0.));
#9086=DIRECTION('ref_axis',(-1.,0.,-1.22464679914735E-16));
#9087=DIRECTION('center_axis',(0.,1.,0.));
#9088=DIRECTION('ref_axis',(1.,0.,0.));
#9089=DIRECTION('center_axis',(0.,1.,0.));
#9090=DIRECTION('ref_axis',(-0.951056516295154,0.,-0.309016994374948));
#9091=DIRECTION('center_axis',(0.,1.,0.));
#9092=DIRECTION('ref_axis',(1.,0.,0.));
#9093=DIRECTION('center_axis',(0.,1.,0.));
#9094=DIRECTION('ref_axis',(-0.809016994374947,0.,-0.587785252292473));
#9095=DIRECTION('center_axis',(0.,1.,0.));
#9096=DIRECTION('ref_axis',(1.,0.,0.));
#9097=DIRECTION('center_axis',(0.,1.,0.));
#9098=DIRECTION('ref_axis',(-0.587785252292473,0.,-0.809016994374948));
#9099=DIRECTION('center_axis',(0.,1.,0.));
#9100=DIRECTION('ref_axis',(1.,0.,0.));
#9101=DIRECTION('center_axis',(0.,1.,0.));
#9102=DIRECTION('ref_axis',(-0.309016994374947,0.,-0.951056516295154));
#9103=DIRECTION('center_axis',(0.,1.,0.));
#9104=DIRECTION('ref_axis',(1.,0.,0.));
#9105=DIRECTION('center_axis',(0.,1.,0.));
#9106=DIRECTION('ref_axis',(6.12323399573677E-17,0.,-1.));
#9107=DIRECTION('center_axis',(0.,1.,0.));
#9108=DIRECTION('ref_axis',(1.,0.,0.));
#9109=DIRECTION('center_axis',(0.,1.,0.));
#9110=DIRECTION('ref_axis',(0.309016994374947,0.,-0.951056516295154));
#9111=DIRECTION('center_axis',(0.,1.,0.));
#9112=DIRECTION('ref_axis',(1.,0.,0.));
#9113=DIRECTION('center_axis',(0.,1.,0.));
#9114=DIRECTION('ref_axis',(0.587785252292473,0.,-0.809016994374947));
#9115=DIRECTION('center_axis',(0.,1.,0.));
#9116=DIRECTION('ref_axis',(1.,0.,0.));
#9117=DIRECTION('center_axis',(0.,1.,0.));
#9118=DIRECTION('ref_axis',(0.809016994374947,0.,-0.587785252292473));
#9119=DIRECTION('center_axis',(0.,1.,0.));
#9120=DIRECTION('ref_axis',(1.,0.,0.));
#9121=DIRECTION('center_axis',(0.,1.,0.));
#9122=DIRECTION('ref_axis',(0.951056516295154,0.,-0.309016994374947));
#9123=DIRECTION('center_axis',(0.,1.,0.));
#9124=DIRECTION('ref_axis',(1.,0.,0.));
#9125=DIRECTION('center_axis',(0.,1.,0.));
#9126=DIRECTION('ref_axis',(1.,0.,0.));
#9127=DIRECTION('center_axis',(0.,1.,0.));
#9128=DIRECTION('ref_axis',(1.,0.,0.));
#9129=DIRECTION('center_axis',(0.,-1.,0.));
#9130=DIRECTION('ref_axis',(1.,0.,0.));
#9131=DIRECTION('center_axis',(0.,-1.,0.));
#9132=DIRECTION('ref_axis',(1.,0.,0.));
#9133=DIRECTION('',(0.,1.,0.));
#9134=DIRECTION('center_axis',(0.,1.,0.));
#9135=DIRECTION('ref_axis',(1.,0.,0.));
#9136=DIRECTION('center_axis',(0.,1.,0.));
#9137=DIRECTION('ref_axis',(1.,0.,0.));
#9138=DIRECTION('center_axis',(0.,1.,0.));
#9139=DIRECTION('ref_axis',(1.,0.,0.));
#9140=DIRECTION('center_axis',(0.,-1.,0.));
#9141=DIRECTION('ref_axis',(0.951056516295154,0.,0.309016994374948));
#9142=DIRECTION('center_axis',(0.,1.,0.));
#9143=DIRECTION('ref_axis',(1.,0.,0.));
#9144=DIRECTION('center_axis',(0.,-1.,0.));
#9145=DIRECTION('ref_axis',(1.,0.,0.));
#9146=DIRECTION('center_axis',(0.,1.,0.));
#9147=DIRECTION('ref_axis',(1.,0.,0.));
#9148=DIRECTION('center_axis',(0.,-1.,0.));
#9149=DIRECTION('ref_axis',(0.951056516295154,0.,-0.309016994374947));
#9150=DIRECTION('center_axis',(0.,1.,0.));
#9151=DIRECTION('ref_axis',(1.,0.,0.));
#9152=DIRECTION('center_axis',(0.,-1.,0.));
#9153=DIRECTION('ref_axis',(0.809016994374947,0.,-0.587785252292473));
#9154=DIRECTION('center_axis',(0.,1.,0.));
#9155=DIRECTION('ref_axis',(1.,0.,0.));
#9156=DIRECTION('center_axis',(0.,-1.,0.));
#9157=DIRECTION('ref_axis',(0.587785252292473,0.,-0.809016994374947));
#9158=DIRECTION('center_axis',(0.,1.,0.));
#9159=DIRECTION('ref_axis',(1.,0.,0.));
#9160=DIRECTION('center_axis',(0.,-1.,0.));
#9161=DIRECTION('ref_axis',(0.309016994374947,0.,-0.951056516295154));
#9162=DIRECTION('center_axis',(0.,1.,0.));
#9163=DIRECTION('ref_axis',(1.,0.,0.));
#9164=DIRECTION('center_axis',(0.,-1.,0.));
#9165=DIRECTION('ref_axis',(6.12323399573677E-17,0.,-1.));
#9166=DIRECTION('center_axis',(0.,1.,0.));
#9167=DIRECTION('ref_axis',(1.,0.,0.));
#9168=DIRECTION('center_axis',(0.,-1.,0.));
#9169=DIRECTION('ref_axis',(-0.309016994374947,0.,-0.951056516295154));
#9170=DIRECTION('center_axis',(0.,1.,0.));
#9171=DIRECTION('ref_axis',(1.,0.,0.));
#9172=DIRECTION('center_axis',(0.,-1.,0.));
#9173=DIRECTION('ref_axis',(-0.587785252292473,0.,-0.809016994374948));
#9174=DIRECTION('center_axis',(0.,1.,0.));
#9175=DIRECTION('ref_axis',(1.,0.,0.));
#9176=DIRECTION('center_axis',(0.,-1.,0.));
#9177=DIRECTION('ref_axis',(-0.809016994374947,0.,-0.587785252292473));
#9178=DIRECTION('center_axis',(0.,1.,0.));
#9179=DIRECTION('ref_axis',(1.,0.,0.));
#9180=DIRECTION('center_axis',(0.,-1.,0.));
#9181=DIRECTION('ref_axis',(-0.951056516295154,0.,-0.309016994374948));
#9182=DIRECTION('center_axis',(0.,1.,0.));
#9183=DIRECTION('ref_axis',(1.,0.,0.));
#9184=DIRECTION('center_axis',(0.,-1.,0.));
#9185=DIRECTION('ref_axis',(-1.,0.,-1.22464679914735E-16));
#9186=DIRECTION('center_axis',(0.,1.,0.));
#9187=DIRECTION('ref_axis',(1.,0.,0.));
#9188=DIRECTION('center_axis',(0.,-1.,0.));
#9189=DIRECTION('ref_axis',(-0.951056516295154,0.,0.309016994374947));
#9190=DIRECTION('center_axis',(0.,1.,0.));
#9191=DIRECTION('ref_axis',(1.,0.,0.));
#9192=DIRECTION('center_axis',(0.,-1.,0.));
#9193=DIRECTION('ref_axis',(-0.809016994374947,0.,0.587785252292473));
#9194=DIRECTION('center_axis',(0.,1.,0.));
#9195=DIRECTION('ref_axis',(1.,0.,0.));
#9196=DIRECTION('center_axis',(0.,-1.,0.));
#9197=DIRECTION('ref_axis',(-0.587785252292473,0.,0.809016994374947));
#9198=DIRECTION('center_axis',(0.,1.,0.));
#9199=DIRECTION('ref_axis',(1.,0.,0.));
#9200=DIRECTION('center_axis',(0.,-1.,0.));
#9201=DIRECTION('ref_axis',(-0.309016994374948,0.,0.951056516295154));
#9202=DIRECTION('center_axis',(0.,1.,0.));
#9203=DIRECTION('ref_axis',(1.,0.,0.));
#9204=DIRECTION('center_axis',(0.,-1.,0.));
#9205=DIRECTION('ref_axis',(-1.83697019872103E-16,0.,1.));
#9206=DIRECTION('center_axis',(0.,1.,0.));
#9207=DIRECTION('ref_axis',(1.,0.,0.));
#9208=DIRECTION('center_axis',(0.,-1.,0.));
#9209=DIRECTION('ref_axis',(0.309016994374947,0.,0.951056516295154));
#9210=DIRECTION('center_axis',(0.,1.,0.));
#9211=DIRECTION('ref_axis',(1.,0.,0.));
#9212=DIRECTION('center_axis',(0.,-1.,0.));
#9213=DIRECTION('ref_axis',(0.587785252292473,0.,0.809016994374948));
#9214=DIRECTION('center_axis',(0.,1.,0.));
#9215=DIRECTION('ref_axis',(1.,0.,0.));
#9216=DIRECTION('center_axis',(0.,-1.,0.));
#9217=DIRECTION('ref_axis',(0.809016994374947,0.,0.587785252292473));
#9218=DIRECTION('center_axis',(0.,1.,0.));
#9219=DIRECTION('ref_axis',(1.,0.,0.));
#9220=DIRECTION('center_axis',(0.,1.,0.));
#9221=DIRECTION('ref_axis',(1.,0.,0.));
#9222=DIRECTION('center_axis',(0.,1.,0.));
#9223=DIRECTION('ref_axis',(1.,0.,0.));
#9224=DIRECTION('',(0.,-1.,0.));
#9225=DIRECTION('center_axis',(0.,1.,0.));
#9226=DIRECTION('ref_axis',(1.,0.,0.));
#9227=DIRECTION('center_axis',(0.,1.,0.));
#9228=DIRECTION('ref_axis',(-0.951056516295153,0.,-0.309016994374948));
#9229=DIRECTION('',(0.,-1.,0.));
#9230=DIRECTION('',(0.,1.,0.));
#9231=DIRECTION('center_axis',(0.,1.,0.));
#9232=DIRECTION('ref_axis',(1.,0.,0.));
#9233=DIRECTION('',(0.,-1.,0.));
#9234=DIRECTION('center_axis',(0.,1.,0.));
#9235=DIRECTION('ref_axis',(-0.809016994374947,0.,-0.587785252292473));
#9236=DIRECTION('',(0.,1.,0.));
#9237=DIRECTION('center_axis',(0.,1.,0.));
#9238=DIRECTION('ref_axis',(1.,0.,0.));
#9239=DIRECTION('',(0.,-1.,0.));
#9240=DIRECTION('center_axis',(0.,1.,0.));
#9241=DIRECTION('ref_axis',(-0.587785252292473,0.,-0.809016994374947));
#9242=DIRECTION('',(0.,1.,0.));
#9243=DIRECTION('center_axis',(0.,1.,0.));
#9244=DIRECTION('ref_axis',(1.,0.,0.));
#9245=DIRECTION('',(0.,-1.,0.));
#9246=DIRECTION('center_axis',(0.,1.,0.));
#9247=DIRECTION('ref_axis',(-0.309016994374947,0.,-0.951056516295154));
#9248=DIRECTION('',(0.,1.,0.));
#9249=DIRECTION('center_axis',(0.,1.,0.));
#9250=DIRECTION('ref_axis',(1.,0.,0.));
#9251=DIRECTION('',(0.,-1.,0.));
#9252=DIRECTION('center_axis',(0.,1.,0.));
#9253=DIRECTION('ref_axis',(-1.37927510063224E-16,0.,-1.));
#9254=DIRECTION('',(0.,1.,0.));
#9255=DIRECTION('center_axis',(0.,1.,0.));
#9256=DIRECTION('ref_axis',(1.,0.,0.));
#9257=DIRECTION('',(0.,-1.,0.));
#9258=DIRECTION('center_axis',(0.,1.,0.));
#9259=DIRECTION('ref_axis',(0.309016994374948,0.,-0.951056516295154));
#9260=DIRECTION('',(0.,1.,0.));
#9261=DIRECTION('center_axis',(0.,1.,0.));
#9262=DIRECTION('ref_axis',(1.,0.,0.));
#9263=DIRECTION('',(0.,-1.,0.));
#9264=DIRECTION('center_axis',(0.,1.,0.));
#9265=DIRECTION('ref_axis',(0.587785252292473,0.,-0.809016994374948));
#9266=DIRECTION('',(0.,1.,0.));
#9267=DIRECTION('center_axis',(0.,1.,0.));
#9268=DIRECTION('ref_axis',(1.,0.,0.));
#9269=DIRECTION('',(0.,-1.,0.));
#9270=DIRECTION('center_axis',(0.,1.,0.));
#9271=DIRECTION('ref_axis',(0.809016994374948,0.,-0.587785252292473));
#9272=DIRECTION('',(0.,1.,0.));
#9273=DIRECTION('center_axis',(0.,1.,0.));
#9274=DIRECTION('ref_axis',(1.,0.,0.));
#9275=DIRECTION('',(0.,-1.,0.));
#9276=DIRECTION('center_axis',(0.,1.,0.));
#9277=DIRECTION('ref_axis',(0.951056516295154,0.,-0.309016994374947));
#9278=DIRECTION('',(0.,1.,0.));
#9279=DIRECTION('center_axis',(0.,1.,0.));
#9280=DIRECTION('ref_axis',(1.,0.,0.));
#9281=DIRECTION('',(0.,-1.,0.));
#9282=DIRECTION('center_axis',(0.,1.,0.));
#9283=DIRECTION('ref_axis',(1.,0.,-1.99159850020592E-16));
#9284=DIRECTION('',(0.,1.,0.));
#9285=DIRECTION('center_axis',(0.,1.,0.));
#9286=DIRECTION('ref_axis',(1.,0.,0.));
#9287=DIRECTION('',(0.,-1.,0.));
#9288=DIRECTION('center_axis',(0.,1.,0.));
#9289=DIRECTION('ref_axis',(0.951056516295154,0.,0.309016994374948));
#9290=DIRECTION('',(0.,1.,0.));
#9291=DIRECTION('center_axis',(0.,1.,0.));
#9292=DIRECTION('ref_axis',(1.,0.,0.));
#9293=DIRECTION('',(0.,-1.,0.));
#9294=DIRECTION('center_axis',(0.,1.,0.));
#9295=DIRECTION('ref_axis',(0.809016994374948,0.,0.587785252292473));
#9296=DIRECTION('',(0.,1.,0.));
#9297=DIRECTION('center_axis',(0.,1.,0.));
#9298=DIRECTION('ref_axis',(1.,0.,0.));
#9299=DIRECTION('',(0.,-1.,0.));
#9300=DIRECTION('center_axis',(0.,1.,0.));
#9301=DIRECTION('ref_axis',(0.587785252292473,0.,0.809016994374948));
#9302=DIRECTION('',(0.,1.,0.));
#9303=DIRECTION('center_axis',(0.,1.,0.));
#9304=DIRECTION('ref_axis',(1.,0.,0.));
#9305=DIRECTION('',(0.,-1.,0.));
#9306=DIRECTION('center_axis',(0.,1.,0.));
#9307=DIRECTION('ref_axis',(0.309016994374947,0.,0.951056516295154));
#9308=DIRECTION('',(0.,1.,0.));
#9309=DIRECTION('center_axis',(0.,1.,0.));
#9310=DIRECTION('ref_axis',(1.,0.,0.));
#9311=DIRECTION('',(0.,-1.,0.));
#9312=DIRECTION('center_axis',(0.,1.,0.));
#9313=DIRECTION('ref_axis',(2.6039218997796E-16,0.,1.));
#9314=DIRECTION('',(0.,1.,0.));
#9315=DIRECTION('center_axis',(0.,1.,0.));
#9316=DIRECTION('ref_axis',(1.,0.,0.));
#9317=DIRECTION('',(0.,-1.,0.));
#9318=DIRECTION('center_axis',(0.,1.,0.));
#9319=DIRECTION('ref_axis',(-0.309016994374948,0.,0.951056516295153));
#9320=DIRECTION('',(0.,1.,0.));
#9321=DIRECTION('center_axis',(0.,1.,0.));
#9322=DIRECTION('ref_axis',(1.,0.,0.));
#9323=DIRECTION('',(0.,-1.,0.));
#9324=DIRECTION('center_axis',(0.,1.,0.));
#9325=DIRECTION('ref_axis',(-0.587785252292474,0.,0.809016994374947));
#9326=DIRECTION('',(0.,1.,0.));
#9327=DIRECTION('center_axis',(0.,1.,0.));
#9328=DIRECTION('ref_axis',(1.,0.,0.));
#9329=DIRECTION('',(0.,-1.,0.));
#9330=DIRECTION('center_axis',(0.,1.,0.));
#9331=DIRECTION('ref_axis',(-0.809016994374948,0.,0.587785252292473));
#9332=DIRECTION('',(0.,1.,0.));
#9333=DIRECTION('center_axis',(0.,1.,0.));
#9334=DIRECTION('ref_axis',(1.,0.,0.));
#9335=DIRECTION('',(0.,-1.,0.));
#9336=DIRECTION('center_axis',(0.,1.,0.));
#9337=DIRECTION('ref_axis',(-0.951056516295154,0.,0.309016994374948));
#9338=DIRECTION('',(0.,1.,0.));
#9339=DIRECTION('center_axis',(0.,1.,0.));
#9340=DIRECTION('ref_axis',(1.,0.,0.));
#9341=DIRECTION('',(0.,1.,0.));
#9342=DIRECTION('center_axis',(0.,1.,0.));
#9343=DIRECTION('ref_axis',(-1.,0.,-1.22464679914735E-16));
#9344=DIRECTION('',(0.,-1.,0.));
#9345=DIRECTION('center_axis',(0.,1.,0.));
#9346=DIRECTION('ref_axis',(1.,0.,0.));
#12019=CARTESIAN_POINT('',(0.,0.,0.));
#12020=CARTESIAN_POINT('Origin',(0.,-0.45,0.));
#12021=CARTESIAN_POINT('',(-0.65,-0.325,-3.9801020972289E-17));
#12022=CARTESIAN_POINT('',(-0.637867541108654,-0.45,0.125));
#12023=CARTESIAN_POINT('Ctrl Pts',(-0.65,-0.325,-6.93889390390723E-17));
#12024=CARTESIAN_POINT('Ctrl Pts',(-0.65,-0.325,0.0157371373481997));
#12025=CARTESIAN_POINT('Ctrl Pts',(-0.649370620646074,-0.328153081062251,
0.0324967135411163));
#12026=CARTESIAN_POINT('Ctrl Pts',(-0.647096224417991,-0.340922081922822,
0.0632828231545122));
#12027=CARTESIAN_POINT('Ctrl Pts',(-0.645482573914132,-0.350535859112198,
0.0773125544088347));
#12028=CARTESIAN_POINT('Ctrl Pts',(-0.642442040715078,-0.372687974598127,
0.0994646698947638));
#12029=CARTESIAN_POINT('Ctrl Pts',(-0.640815160902589,-0.386717480603274,
0.109078032552995));
#12030=CARTESIAN_POINT('Ctrl Pts',(-0.63851034608138,-0.417502809542363,
0.121846732641678));
#12031=CARTESIAN_POINT('Ctrl Pts',(-0.637867541108654,-0.434262111007648,
0.125));
#12032=CARTESIAN_POINT('Ctrl Pts',(-0.637867541108654,-0.45,0.125));
#12033=CARTESIAN_POINT('',(-0.65,-0.575,-3.9801020972289E-17));
#12034=CARTESIAN_POINT('Ctrl Pts',(-0.65,-0.575,-3.46944695195361E-18));
#12035=CARTESIAN_POINT('Ctrl Pts',(-0.65,-0.575,-0.0157371373481998));
#12036=CARTESIAN_POINT('Ctrl Pts',(-0.649370620646074,-0.571846918937749,
-0.0324967135411164));
#12037=CARTESIAN_POINT('Ctrl Pts',(-0.647096224417991,-0.559077918077178,
-0.0632828231545123));
#12038=CARTESIAN_POINT('Ctrl Pts',(-0.645482573914132,-0.549464140887802,
-0.0773125544088349));
#12039=CARTESIAN_POINT('Ctrl Pts',(-0.642442040715078,-0.527312025401873,
-0.099464669894764));
#12040=CARTESIAN_POINT('Ctrl Pts',(-0.640815160902589,-0.513282519396725,
-0.109078032552995));
#12041=CARTESIAN_POINT('Ctrl Pts',(-0.63851034608138,-0.482497190457637,
-0.121846732641678));
#12042=CARTESIAN_POINT('Ctrl Pts',(-0.637867541108654,-0.465737888992352,
-0.125));
#12043=CARTESIAN_POINT('Ctrl Pts',(-0.637867541108654,-0.434262111007648,
-0.125));
#12044=CARTESIAN_POINT('Ctrl Pts',(-0.63851034608138,-0.417502809542363,
-0.121846732641678));
#12045=CARTESIAN_POINT('Ctrl Pts',(-0.640815160902589,-0.386717480603275,
-0.109078032552995));
#12046=CARTESIAN_POINT('Ctrl Pts',(-0.642442040715078,-0.372687974598127,
-0.099464669894764));
#12047=CARTESIAN_POINT('Ctrl Pts',(-0.645482573914132,-0.350535859112198,
-0.077312554408835));
#12048=CARTESIAN_POINT('Ctrl Pts',(-0.647096224417991,-0.340922081922822,
-0.0632828231545124));
#12049=CARTESIAN_POINT('Ctrl Pts',(-0.649370620646074,-0.328153081062251,
-0.0324967135411165));
#12050=CARTESIAN_POINT('Ctrl Pts',(-0.65,-0.325,-0.0157371373481999));
#12051=CARTESIAN_POINT('Ctrl Pts',(-0.65,-0.325,-8.32667268468867E-17));
#12052=CARTESIAN_POINT('Ctrl Pts',(-0.637867541108654,-0.45,0.125));
#12053=CARTESIAN_POINT('Ctrl Pts',(-0.637867541108654,-0.465737888992352,
0.125));
#12054=CARTESIAN_POINT('Ctrl Pts',(-0.63851034608138,-0.482497190457637,
0.121846732641678));
#12055=CARTESIAN_POINT('Ctrl Pts',(-0.640815160902589,-0.513282519396725,
0.109078032552995));
#12056=CARTESIAN_POINT('Ctrl Pts',(-0.642442040715078,-0.527312025401873,
0.0994646698947639));
#12057=CARTESIAN_POINT('Ctrl Pts',(-0.645482573914132,-0.549464140887802,
0.0773125544088349));
#12058=CARTESIAN_POINT('Ctrl Pts',(-0.647096224417991,-0.559077918077178,
0.0632828231545123));
#12059=CARTESIAN_POINT('Ctrl Pts',(-0.649370620646074,-0.571846918937749,
0.0324967135411164));
#12060=CARTESIAN_POINT('Ctrl Pts',(-0.65,-0.575,0.0157371373481998));
#12061=CARTESIAN_POINT('Ctrl Pts',(-0.65,-0.575,-2.08166817117217E-17));
#12062=CARTESIAN_POINT('',(-0.379967103839267,-0.45,0.125));
#12063=CARTESIAN_POINT('',(-7.65404249467096E-18,-0.45,0.125));
#12064=CARTESIAN_POINT('',(-0.4,-0.575,5.41097774720219E-18));
#12065=CARTESIAN_POINT('Ctrl Pts',(-0.4,-0.575,-3.81639164714898E-17));
#12066=CARTESIAN_POINT('Ctrl Pts',(-0.4,-0.575,0.0158075115832675));
#12067=CARTESIAN_POINT('Ctrl Pts',(-0.398970551469948,-0.571819306519379,
0.0325978607437828));
#12068=CARTESIAN_POINT('Ctrl Pts',(-0.395252954914593,-0.559029081159106,
0.0633657881355917));
#12069=CARTESIAN_POINT('Ctrl Pts',(-0.392612801026882,-0.549425200318011,
0.0773514949786256));
#12070=CARTESIAN_POINT('Ctrl Pts',(-0.38761064154154,-0.527347592689753,
0.0994291026068839));
#12071=CARTESIAN_POINT('Ctrl Pts',(-0.384911758361269,-0.51336346023721,
0.109029967924066));
#12072=CARTESIAN_POINT('Ctrl Pts',(-0.381057715344782,-0.48260129709332,
0.121817958968287));
#12073=CARTESIAN_POINT('Ctrl Pts',(-0.379967103839267,-0.465813100629203,
0.125));
#12074=CARTESIAN_POINT('Ctrl Pts',(-0.379967103839267,-0.45,0.125));
#12075=CARTESIAN_POINT('',(-0.379967103839267,-0.45,-0.125));
#12076=CARTESIAN_POINT('Ctrl Pts',(-0.379967103839267,-0.45,-0.125));
#12077=CARTESIAN_POINT('Ctrl Pts',(-0.379967103839267,-0.465813100629203,
-0.125));
#12078=CARTESIAN_POINT('Ctrl Pts',(-0.381057715344782,-0.48260129709332,
-0.121817958968287));
#12079=CARTESIAN_POINT('Ctrl Pts',(-0.384911758361269,-0.51336346023721,
-0.109029967924066));
#12080=CARTESIAN_POINT('Ctrl Pts',(-0.38761064154154,-0.527347592689753,
-0.099429102606884));
#12081=CARTESIAN_POINT('Ctrl Pts',(-0.392612801026882,-0.549425200318011,
-0.0773514949786257));
#12082=CARTESIAN_POINT('Ctrl Pts',(-0.395252954914593,-0.559029081159106,
-0.0633657881355918));
#12083=CARTESIAN_POINT('Ctrl Pts',(-0.398970551469948,-0.571819306519379,
-0.0325978607437828));
#12084=CARTESIAN_POINT('Ctrl Pts',(-0.4,-0.575,-0.0158075115832676));
#12085=CARTESIAN_POINT('Ctrl Pts',(-0.4,-0.575,-4.16333634234434E-17));
#12086=CARTESIAN_POINT('',(-0.4,-0.325,2.96971064108775E-17));
#12087=CARTESIAN_POINT('Ctrl Pts',(-0.4,-0.325,1.04083408558608E-17));
#12088=CARTESIAN_POINT('Ctrl Pts',(-0.4,-0.325,-0.0158075115832676));
#12089=CARTESIAN_POINT('Ctrl Pts',(-0.398970551469948,-0.328180693480621,
-0.0325978607437828));
#12090=CARTESIAN_POINT('Ctrl Pts',(-0.395252954914593,-0.340970918840894,
-0.0633657881355918));
#12091=CARTESIAN_POINT('Ctrl Pts',(-0.392612801026882,-0.350574799681989,
-0.0773514949786256));
#12092=CARTESIAN_POINT('Ctrl Pts',(-0.38761064154154,-0.372652407310247,
-0.0994291026068839));
#12093=CARTESIAN_POINT('Ctrl Pts',(-0.384911758361269,-0.38663653976279,
-0.109029967924066));
#12094=CARTESIAN_POINT('Ctrl Pts',(-0.381057715344782,-0.41739870290668,
-0.121817958968287));
#12095=CARTESIAN_POINT('Ctrl Pts',(-0.379967103839267,-0.434186899370797,
-0.125));
#12096=CARTESIAN_POINT('Ctrl Pts',(-0.379967103839267,-0.45,-0.125));
#12097=CARTESIAN_POINT('Ctrl Pts',(-0.379967103839267,-0.45,0.125));
#12098=CARTESIAN_POINT('Ctrl Pts',(-0.379967103839267,-0.434186899370797,
0.125));
#12099=CARTESIAN_POINT('Ctrl Pts',(-0.381057715344782,-0.41739870290668,
0.121817958968287));
#12100=CARTESIAN_POINT('Ctrl Pts',(-0.384911758361269,-0.38663653976279,
0.109029967924066));
#12101=CARTESIAN_POINT('Ctrl Pts',(-0.38761064154154,-0.372652407310247,
0.0994291026068839));
#12102=CARTESIAN_POINT('Ctrl Pts',(-0.392612801026882,-0.350574799681989,
0.0773514949786257));
#12103=CARTESIAN_POINT('Ctrl Pts',(-0.395252954914593,-0.340970918840894,
0.0633657881355918));
#12104=CARTESIAN_POINT('Ctrl Pts',(-0.398970551469948,-0.328180693480621,
0.0325978607437829));
#12105=CARTESIAN_POINT('Ctrl Pts',(-0.4,-0.325,0.0158075115832676));
#12106=CARTESIAN_POINT('Ctrl Pts',(-0.4,-0.325,1.38777878078145E-17));
#12107=CARTESIAN_POINT('Origin',(0.,-0.45,0.));
#12108=CARTESIAN_POINT('',(0.379967103839267,-0.45,-0.125));
#12109=CARTESIAN_POINT('',(0.379967103839267,-0.45,0.125));
#12110=CARTESIAN_POINT('Ctrl Pts',(0.379967103839267,-0.45,-0.125));
#12111=CARTESIAN_POINT('Ctrl Pts',(0.379967103839267,-0.434186899370797,
-0.125));
#12112=CARTESIAN_POINT('Ctrl Pts',(0.381057715344782,-0.41739870290668,
-0.121817958968287));
#12113=CARTESIAN_POINT('Ctrl Pts',(0.384911758361269,-0.38663653976279,
-0.109029967924066));
#12114=CARTESIAN_POINT('Ctrl Pts',(0.38761064154154,-0.372652407310247,
-0.0994291026068839));
#12115=CARTESIAN_POINT('Ctrl Pts',(0.392612801026882,-0.350574799681989,
-0.0773514949786256));
#12116=CARTESIAN_POINT('Ctrl Pts',(0.395252954914593,-0.340970918840894,
-0.0633657881355917));
#12117=CARTESIAN_POINT('Ctrl Pts',(0.398970551469948,-0.328180693480621,
-0.0325978607437828));
#12118=CARTESIAN_POINT('Ctrl Pts',(0.4,-0.325,-0.0158075115832675));
#12119=CARTESIAN_POINT('Ctrl Pts',(0.4,-0.325,0.0158075115832676));
#12120=CARTESIAN_POINT('Ctrl Pts',(0.398970551469948,-0.328180693480621,
0.0325978607437829));
#12121=CARTESIAN_POINT('Ctrl Pts',(0.395252954914593,-0.340970918840894,
0.0633657881355918));
#12122=CARTESIAN_POINT('Ctrl Pts',(0.392612801026882,-0.350574799681989,
0.0773514949786257));
#12123=CARTESIAN_POINT('Ctrl Pts',(0.38761064154154,-0.372652407310247,
0.099429102606884));
#12124=CARTESIAN_POINT('Ctrl Pts',(0.384911758361269,-0.38663653976279,
0.109029967924066));
#12125=CARTESIAN_POINT('Ctrl Pts',(0.381057715344782,-0.41739870290668,
0.121817958968287));
#12126=CARTESIAN_POINT('Ctrl Pts',(0.379967103839267,-0.434186899370797,
0.125));
#12127=CARTESIAN_POINT('Ctrl Pts',(0.379967103839267,-0.45,0.125));
#12128=CARTESIAN_POINT('Ctrl Pts',(0.379967103839267,-0.45,0.125));
#12129=CARTESIAN_POINT('Ctrl Pts',(0.379967103839267,-0.465813100629203,
0.125));
#12130=CARTESIAN_POINT('Ctrl Pts',(0.381057715344782,-0.48260129709332,
0.121817958968287));
#12131=CARTESIAN_POINT('Ctrl Pts',(0.384911758361269,-0.51336346023721,
0.109029967924066));
#12132=CARTESIAN_POINT('Ctrl Pts',(0.38761064154154,-0.527347592689753,
0.0994291026068839));
#12133=CARTESIAN_POINT('Ctrl Pts',(0.392612801026882,-0.549425200318011,
0.0773514949786257));
#12134=CARTESIAN_POINT('Ctrl Pts',(0.395252954914593,-0.559029081159106,
0.0633657881355918));
#12135=CARTESIAN_POINT('Ctrl Pts',(0.398970551469948,-0.571819306519379,
0.0325978607437829));
#12136=CARTESIAN_POINT('Ctrl Pts',(0.4,-0.575,0.0158075115832676));
#12137=CARTESIAN_POINT('Ctrl Pts',(0.4,-0.575,-0.0158075115832676));
#12138=CARTESIAN_POINT('Ctrl Pts',(0.398970551469948,-0.57181930651938,
-0.0325978607437828));
#12139=CARTESIAN_POINT('Ctrl Pts',(0.395252954914593,-0.559029081159106,
-0.0633657881355918));
#12140=CARTESIAN_POINT('Ctrl Pts',(0.392612801026882,-0.549425200318011,
-0.0773514949786257));
#12141=CARTESIAN_POINT('Ctrl Pts',(0.38761064154154,-0.527347592689753,
-0.0994291026068839));
#12142=CARTESIAN_POINT('Ctrl Pts',(0.384911758361269,-0.51336346023721,
-0.109029967924066));
#12143=CARTESIAN_POINT('Ctrl Pts',(0.381057715344782,-0.48260129709332,
-0.121817958968287));
#12144=CARTESIAN_POINT('Ctrl Pts',(0.379967103839267,-0.465813100629203,
-0.125));
#12145=CARTESIAN_POINT('Ctrl Pts',(0.379967103839267,-0.45,-0.125));
#12146=CARTESIAN_POINT('',(0.637867541108654,-0.45,0.125));
#12147=CARTESIAN_POINT('',(-7.65404249467096E-18,-0.45,0.125));
#12148=CARTESIAN_POINT('',(0.65,-0.575,3.9801020972289E-17));
#12149=CARTESIAN_POINT('Ctrl Pts',(0.65,-0.575,5.55111512312578E-17));
#12150=CARTESIAN_POINT('Ctrl Pts',(0.65,-0.575,0.0157371373481999));
#12151=CARTESIAN_POINT('Ctrl Pts',(0.649370620646074,-0.571846918937749,
0.0324967135411165));
#12152=CARTESIAN_POINT('Ctrl Pts',(0.647096224417991,-0.559077918077178,
0.0632828231545124));
#12153=CARTESIAN_POINT('Ctrl Pts',(0.645482573914132,-0.549464140887802,
0.077312554408835));
#12154=CARTESIAN_POINT('Ctrl Pts',(0.642442040715078,-0.527312025401873,
0.099464669894764));
#12155=CARTESIAN_POINT('Ctrl Pts',(0.640815160902589,-0.513282519396725,
0.109078032552995));
#12156=CARTESIAN_POINT('Ctrl Pts',(0.63851034608138,-0.482497190457637,
0.121846732641678));
#12157=CARTESIAN_POINT('Ctrl Pts',(0.637867541108654,-0.465737888992352,
0.125));
#12158=CARTESIAN_POINT('Ctrl Pts',(0.637867541108654,-0.45,0.125));
#12159=CARTESIAN_POINT('',(0.65,-0.325,3.9801020972289E-17));
#12160=CARTESIAN_POINT('Ctrl Pts',(0.65,-0.325,6.93889390390723E-18));
#12161=CARTESIAN_POINT('Ctrl Pts',(0.65,-0.325,-0.0157371373481998));
#12162=CARTESIAN_POINT('Ctrl Pts',(0.649370620646074,-0.328153081062251,
-0.0324967135411164));
#12163=CARTESIAN_POINT('Ctrl Pts',(0.647096224417991,-0.340922081922822,
-0.0632828231545123));
#12164=CARTESIAN_POINT('Ctrl Pts',(0.645482573914132,-0.350535859112198,
-0.0773125544088349));
#12165=CARTESIAN_POINT('Ctrl Pts',(0.642442040715078,-0.372687974598127,
-0.0994646698947639));
#12166=CARTESIAN_POINT('Ctrl Pts',(0.640815160902588,-0.386717480603275,
-0.109078032552995));
#12167=CARTESIAN_POINT('Ctrl Pts',(0.63851034608138,-0.417502809542363,
-0.121846732641678));
#12168=CARTESIAN_POINT('Ctrl Pts',(0.637867541108654,-0.434262111007648,
-0.125));
#12169=CARTESIAN_POINT('Ctrl Pts',(0.637867541108654,-0.465737888992352,
-0.125));
#12170=CARTESIAN_POINT('Ctrl Pts',(0.63851034608138,-0.482497190457637,
-0.121846732641678));
#12171=CARTESIAN_POINT('Ctrl Pts',(0.640815160902589,-0.513282519396725,
-0.109078032552995));
#12172=CARTESIAN_POINT('Ctrl Pts',(0.642442040715078,-0.527312025401873,
-0.0994646698947639));
#12173=CARTESIAN_POINT('Ctrl Pts',(0.645482573914132,-0.549464140887802,
-0.0773125544088348));
#12174=CARTESIAN_POINT('Ctrl Pts',(0.647096224417991,-0.559077918077178,
-0.0632828231545123));
#12175=CARTESIAN_POINT('Ctrl Pts',(0.649370620646074,-0.571846918937749,
-0.0324967135411164));
#12176=CARTESIAN_POINT('Ctrl Pts',(0.65,-0.575,-0.0157371373481998));
#12177=CARTESIAN_POINT('Ctrl Pts',(0.65,-0.575,6.24500451351651E-17));
#12178=CARTESIAN_POINT('Ctrl Pts',(0.637867541108654,-0.45,0.125));
#12179=CARTESIAN_POINT('Ctrl Pts',(0.637867541108654,-0.434262111007648,
0.125));
#12180=CARTESIAN_POINT('Ctrl Pts',(0.63851034608138,-0.417502809542363,
0.121846732641678));
#12181=CARTESIAN_POINT('Ctrl Pts',(0.640815160902589,-0.386717480603274,
0.109078032552995));
#12182=CARTESIAN_POINT('Ctrl Pts',(0.642442040715078,-0.372687974598127,
0.0994646698947639));
#12183=CARTESIAN_POINT('Ctrl Pts',(0.645482573914132,-0.350535859112198,
0.0773125544088348));
#12184=CARTESIAN_POINT('Ctrl Pts',(0.647096224417991,-0.340922081922822,
0.0632828231545123));
#12185=CARTESIAN_POINT('Ctrl Pts',(0.649370620646074,-0.328153081062251,
0.0324967135411164));
#12186=CARTESIAN_POINT('Ctrl Pts',(0.65,-0.325,0.0157371373481998));
#12187=CARTESIAN_POINT('Ctrl Pts',(0.65,-0.325,-6.93889390390723E-18));
#12188=CARTESIAN_POINT('Origin',(0.,-0.1,0.));
#12189=CARTESIAN_POINT('',(-0.65,-0.8,7.9602041944578E-17));
#12190=CARTESIAN_POINT('Origin',(0.,-0.8,0.));
#12191=CARTESIAN_POINT('',(-0.65,-0.1,-7.9602041944578E-17));
#12192=CARTESIAN_POINT('',(-0.65,-0.1,7.9602041944578E-17));
#12193=CARTESIAN_POINT('',(-0.65,-0.1,-7.9602041944578E-17));
#12194=CARTESIAN_POINT('Origin',(0.,-0.1,0.));
#12195=CARTESIAN_POINT('',(0.,-0.575,-0.65));
#12196=CARTESIAN_POINT('',(0.,-0.325,-0.65));
#12197=CARTESIAN_POINT('Ctrl Pts',(-1.73472347597681E-17,-0.575,-0.65));
#12198=CARTESIAN_POINT('Ctrl Pts',(0.0157371373481998,-0.575,-0.65));
#12199=CARTESIAN_POINT('Ctrl Pts',(0.0324967135411164,-0.571846918937749,
-0.649370620646074));
#12200=CARTESIAN_POINT('Ctrl Pts',(0.0632828231545123,-0.559077918077178,
-0.647096224417991));
#12201=CARTESIAN_POINT('Ctrl Pts',(0.0773125544088349,-0.549464140887802,
-0.645482573914132));
#12202=CARTESIAN_POINT('Ctrl Pts',(0.099464669894764,-0.527312025401873,
-0.642442040715078));
#12203=CARTESIAN_POINT('Ctrl Pts',(0.109078032552995,-0.513282519396725,
-0.640815160902589));
#12204=CARTESIAN_POINT('Ctrl Pts',(0.121846732641678,-0.482497190457636,
-0.63851034608138));
#12205=CARTESIAN_POINT('Ctrl Pts',(0.125,-0.465737888992352,-0.637867541108654));
#12206=CARTESIAN_POINT('Ctrl Pts',(0.125,-0.434262111007648,-0.637867541108654));
#12207=CARTESIAN_POINT('Ctrl Pts',(0.121846732641678,-0.417502809542364,
-0.63851034608138));
#12208=CARTESIAN_POINT('Ctrl Pts',(0.109078032552995,-0.386717480603275,
-0.640815160902589));
#12209=CARTESIAN_POINT('Ctrl Pts',(0.099464669894764,-0.372687974598127,
-0.642442040715078));
#12210=CARTESIAN_POINT('Ctrl Pts',(0.0773125544088349,-0.350535859112198,
-0.645482573914132));
#12211=CARTESIAN_POINT('Ctrl Pts',(0.0632828231545123,-0.340922081922822,
-0.647096224417991));
#12212=CARTESIAN_POINT('Ctrl Pts',(0.0324967135411164,-0.328153081062251,
-0.649370620646074));
#12213=CARTESIAN_POINT('Ctrl Pts',(0.0157371373481999,-0.325,-0.65));
#12214=CARTESIAN_POINT('Ctrl Pts',(4.5102810375397E-17,-0.325,-0.65));
#12215=CARTESIAN_POINT('',(-0.125,-0.45,-0.637867541108654));
#12216=CARTESIAN_POINT('Ctrl Pts',(4.85722573273506E-17,-0.325,-0.65));
#12217=CARTESIAN_POINT('Ctrl Pts',(-0.0157371373481997,-0.325,-0.65));
#12218=CARTESIAN_POINT('Ctrl Pts',(-0.0324967135411163,-0.328153081062251,
-0.649370620646074));
#12219=CARTESIAN_POINT('Ctrl Pts',(-0.0632828231545122,-0.340922081922822,
-0.647096224417991));
#12220=CARTESIAN_POINT('Ctrl Pts',(-0.0773125544088348,-0.350535859112198,
-0.645482573914132));
#12221=CARTESIAN_POINT('Ctrl Pts',(-0.0994646698947639,-0.372687974598127,
-0.642442040715078));
#12222=CARTESIAN_POINT('Ctrl Pts',(-0.109078032552995,-0.386717480603274,
-0.640815160902589));
#12223=CARTESIAN_POINT('Ctrl Pts',(-0.121846732641678,-0.417502809542363,
-0.63851034608138));
#12224=CARTESIAN_POINT('Ctrl Pts',(-0.125,-0.434262111007648,-0.637867541108654));
#12225=CARTESIAN_POINT('Ctrl Pts',(-0.125,-0.45,-0.637867541108654));
#12226=CARTESIAN_POINT('Ctrl Pts',(-0.125,-0.45,-0.637867541108654));
#12227=CARTESIAN_POINT('Ctrl Pts',(-0.125,-0.465737888992352,-0.637867541108654));
#12228=CARTESIAN_POINT('Ctrl Pts',(-0.121846732641678,-0.482497190457636,
-0.63851034608138));
#12229=CARTESIAN_POINT('Ctrl Pts',(-0.109078032552995,-0.513282519396725,
-0.640815160902589));
#12230=CARTESIAN_POINT('Ctrl Pts',(-0.099464669894764,-0.527312025401873,
-0.642442040715078));
#12231=CARTESIAN_POINT('Ctrl Pts',(-0.0773125544088349,-0.549464140887802,
-0.645482573914132));
#12232=CARTESIAN_POINT('Ctrl Pts',(-0.0632828231545124,-0.559077918077178,
-0.647096224417991));
#12233=CARTESIAN_POINT('Ctrl Pts',(-0.0324967135411165,-0.571846918937749,
-0.649370620646074));
#12234=CARTESIAN_POINT('Ctrl Pts',(-0.0157371373481998,-0.575,-0.65));
#12235=CARTESIAN_POINT('Ctrl Pts',(-1.73472347597681E-17,-0.575,-0.65));
#12236=CARTESIAN_POINT('',(0.,-0.325,0.65));
#12237=CARTESIAN_POINT('',(0.,-0.575,0.65));
#12238=CARTESIAN_POINT('Ctrl Pts',(2.77555756156289E-17,-0.325,0.65));
#12239=CARTESIAN_POINT('Ctrl Pts',(0.0157371373481998,-0.325,0.65));
#12240=CARTESIAN_POINT('Ctrl Pts',(0.0324967135411164,-0.328153081062251,
0.649370620646074));
#12241=CARTESIAN_POINT('Ctrl Pts',(0.0632828231545123,-0.340922081922822,
0.647096224417991));
#12242=CARTESIAN_POINT('Ctrl Pts',(0.0773125544088349,-0.350535859112198,
0.645482573914132));
#12243=CARTESIAN_POINT('Ctrl Pts',(0.099464669894764,-0.372687974598127,
0.642442040715078));
#12244=CARTESIAN_POINT('Ctrl Pts',(0.109078032552995,-0.386717480603275,
0.640815160902589));
#12245=CARTESIAN_POINT('Ctrl Pts',(0.121846732641678,-0.417502809542364,
0.63851034608138));
#12246=CARTESIAN_POINT('Ctrl Pts',(0.125,-0.434262111007648,0.637867541108654));
#12247=CARTESIAN_POINT('Ctrl Pts',(0.125,-0.465737888992352,0.637867541108654));
#12248=CARTESIAN_POINT('Ctrl Pts',(0.121846732641678,-0.482497190457636,
0.63851034608138));
#12249=CARTESIAN_POINT('Ctrl Pts',(0.109078032552995,-0.513282519396725,
0.640815160902589));
#12250=CARTESIAN_POINT('Ctrl Pts',(0.099464669894764,-0.527312025401873,
0.642442040715078));
#12251=CARTESIAN_POINT('Ctrl Pts',(0.077312554408835,-0.549464140887802,
0.645482573914132));
#12252=CARTESIAN_POINT('Ctrl Pts',(0.0632828231545124,-0.559077918077178,
0.647096224417991));
#12253=CARTESIAN_POINT('Ctrl Pts',(0.0324967135411165,-0.571846918937749,
0.649370620646074));
#12254=CARTESIAN_POINT('Ctrl Pts',(0.0157371373481998,-0.575,0.65));
#12255=CARTESIAN_POINT('Ctrl Pts',(-1.38777878078145E-17,-0.575,0.65));
#12256=CARTESIAN_POINT('',(-0.125,-0.45,0.637867541108654));
#12257=CARTESIAN_POINT('Ctrl Pts',(-1.04083408558608E-17,-0.575,0.65));
#12258=CARTESIAN_POINT('Ctrl Pts',(-0.0157371373481998,-0.575,0.65));
#12259=CARTESIAN_POINT('Ctrl Pts',(-0.0324967135411164,-0.571846918937749,
0.649370620646074));
#12260=CARTESIAN_POINT('Ctrl Pts',(-0.0632828231545123,-0.559077918077178,
0.647096224417991));
#12261=CARTESIAN_POINT('Ctrl Pts',(-0.0773125544088349,-0.549464140887802,
0.645482573914132));
#12262=CARTESIAN_POINT('Ctrl Pts',(-0.099464669894764,-0.527312025401873,
0.642442040715078));
#12263=CARTESIAN_POINT('Ctrl Pts',(-0.109078032552995,-0.513282519396725,
0.640815160902589));
#12264=CARTESIAN_POINT('Ctrl Pts',(-0.121846732641678,-0.482497190457636,
0.63851034608138));
#12265=CARTESIAN_POINT('Ctrl Pts',(-0.125,-0.465737888992352,0.637867541108654));
#12266=CARTESIAN_POINT('Ctrl Pts',(-0.125,-0.45,0.637867541108654));
#12267=CARTESIAN_POINT('Ctrl Pts',(-0.125,-0.45,0.637867541108654));
#12268=CARTESIAN_POINT('Ctrl Pts',(-0.125,-0.434262111007648,0.637867541108654));
#12269=CARTESIAN_POINT('Ctrl Pts',(-0.121846732641678,-0.417502809542363,
0.63851034608138));
#12270=CARTESIAN_POINT('Ctrl Pts',(-0.109078032552995,-0.386717480603274,
0.640815160902589));
#12271=CARTESIAN_POINT('Ctrl Pts',(-0.0994646698947639,-0.372687974598127,
0.642442040715078));
#12272=CARTESIAN_POINT('Ctrl Pts',(-0.0773125544088348,-0.350535859112198,
0.645482573914132));
#12273=CARTESIAN_POINT('Ctrl Pts',(-0.0632828231545122,-0.340922081922822,
0.647096224417991));
#12274=CARTESIAN_POINT('Ctrl Pts',(-0.0324967135411163,-0.328153081062251,
0.649370620646074));
#12275=CARTESIAN_POINT('Ctrl Pts',(-0.0157371373481998,-0.325,0.65));
#12276=CARTESIAN_POINT('Ctrl Pts',(4.5102810375397E-17,-0.325,0.65));
#12277=CARTESIAN_POINT('Origin',(0.,-0.45,0.));
#12278=CARTESIAN_POINT('',(-0.125,-0.45,-0.379967103839267));
#12279=CARTESIAN_POINT('',(-0.125,-0.45,0.));
#12280=CARTESIAN_POINT('',(0.125,-0.45,-0.379967103839267));
#12281=CARTESIAN_POINT('Ctrl Pts',(0.125,-0.45,-0.379967103839267));
#12282=CARTESIAN_POINT('Ctrl Pts',(0.125,-0.465813100629203,-0.379967103839267));
#12283=CARTESIAN_POINT('Ctrl Pts',(0.121817958968287,-0.48260129709332,
-0.381057715344782));
#12284=CARTESIAN_POINT('Ctrl Pts',(0.109029967924066,-0.51336346023721,
-0.384911758361269));
#12285=CARTESIAN_POINT('Ctrl Pts',(0.0994291026068839,-0.527347592689753,
-0.38761064154154));
#12286=CARTESIAN_POINT('Ctrl Pts',(0.0773514949786257,-0.549425200318011,
-0.392612801026882));
#12287=CARTESIAN_POINT('Ctrl Pts',(0.0633657881355918,-0.559029081159106,
-0.395252954914593));
#12288=CARTESIAN_POINT('Ctrl Pts',(0.0325978607437828,-0.571819306519379,
-0.398970551469948));
#12289=CARTESIAN_POINT('Ctrl Pts',(0.0158075115832676,-0.575,-0.4));
#12290=CARTESIAN_POINT('Ctrl Pts',(-0.0158075115832676,-0.575,-0.4));
#12291=CARTESIAN_POINT('Ctrl Pts',(-0.0325978607437828,-0.571819306519379,
-0.398970551469948));
#12292=CARTESIAN_POINT('Ctrl Pts',(-0.0633657881355918,-0.559029081159106,
-0.395252954914593));
#12293=CARTESIAN_POINT('Ctrl Pts',(-0.0773514949786256,-0.549425200318011,
-0.392612801026882));
#12294=CARTESIAN_POINT('Ctrl Pts',(-0.0994291026068839,-0.527347592689753,
-0.38761064154154));
#12295=CARTESIAN_POINT('Ctrl Pts',(-0.109029967924066,-0.51336346023721,
-0.384911758361269));
#12296=CARTESIAN_POINT('Ctrl Pts',(-0.121817958968287,-0.48260129709332,
-0.381057715344782));
#12297=CARTESIAN_POINT('Ctrl Pts',(-0.125,-0.465813100629203,-0.379967103839267));
#12298=CARTESIAN_POINT('Ctrl Pts',(-0.125,-0.45,-0.379967103839267));
#12299=CARTESIAN_POINT('Ctrl Pts',(-0.125,-0.45,-0.379967103839267));
#12300=CARTESIAN_POINT('Ctrl Pts',(-0.125,-0.434186899370797,-0.379967103839267));
#12301=CARTESIAN_POINT('Ctrl Pts',(-0.121817958968287,-0.41739870290668,
-0.381057715344782));
#12302=CARTESIAN_POINT('Ctrl Pts',(-0.109029967924066,-0.38663653976279,
-0.384911758361269));
#12303=CARTESIAN_POINT('Ctrl Pts',(-0.0994291026068839,-0.372652407310247,
-0.38761064154154));
#12304=CARTESIAN_POINT('Ctrl Pts',(-0.0773514949786257,-0.350574799681989,
-0.392612801026882));
#12305=CARTESIAN_POINT('Ctrl Pts',(-0.0633657881355918,-0.340970918840894,
-0.395252954914593));
#12306=CARTESIAN_POINT('Ctrl Pts',(-0.0325978607437829,-0.328180693480621,
-0.398970551469948));
#12307=CARTESIAN_POINT('Ctrl Pts',(-0.0158075115832676,-0.325,-0.4));
#12308=CARTESIAN_POINT('Ctrl Pts',(0.0158075115832675,-0.325,-0.4));
#12309=CARTESIAN_POINT('Ctrl Pts',(0.0325978607437828,-0.328180693480621,
-0.398970551469948));
#12310=CARTESIAN_POINT('Ctrl Pts',(0.0633657881355917,-0.340970918840894,
-0.395252954914593));
#12311=CARTESIAN_POINT('Ctrl Pts',(0.0773514949786256,-0.350574799681989,
-0.392612801026882));
#12312=CARTESIAN_POINT('Ctrl Pts',(0.0994291026068839,-0.372652407310247,
-0.38761064154154));
#12313=CARTESIAN_POINT('Ctrl Pts',(0.109029967924066,-0.38663653976279,
-0.384911758361269));
#12314=CARTESIAN_POINT('Ctrl Pts',(0.121817958968287,-0.41739870290668,
-0.381057715344782));
#12315=CARTESIAN_POINT('Ctrl Pts',(0.125,-0.434186899370797,-0.379967103839267));
#12316=CARTESIAN_POINT('Ctrl Pts',(0.125,-0.45,-0.379967103839267));
#12317=CARTESIAN_POINT('Origin',(0.,-0.45,0.));
#12318=CARTESIAN_POINT('',(0.125,-0.45,0.379967103839267));
#12319=CARTESIAN_POINT('',(-0.125,-0.45,0.379967103839267));
#12320=CARTESIAN_POINT('Ctrl Pts',(0.125,-0.45,0.379967103839267));
#12321=CARTESIAN_POINT('Ctrl Pts',(0.125,-0.434186899370797,0.379967103839267));
#12322=CARTESIAN_POINT('Ctrl Pts',(0.121817958968287,-0.41739870290668,
0.381057715344782));
#12323=CARTESIAN_POINT('Ctrl Pts',(0.109029967924066,-0.38663653976279,
0.384911758361269));
#12324=CARTESIAN_POINT('Ctrl Pts',(0.0994291026068839,-0.372652407310247,
0.38761064154154));
#12325=CARTESIAN_POINT('Ctrl Pts',(0.0773514949786256,-0.350574799681989,
0.392612801026882));
#12326=CARTESIAN_POINT('Ctrl Pts',(0.0633657881355918,-0.340970918840894,
0.395252954914593));
#12327=CARTESIAN_POINT('Ctrl Pts',(0.0325978607437828,-0.328180693480621,
0.398970551469948));
#12328=CARTESIAN_POINT('Ctrl Pts',(0.0158075115832676,-0.325,0.4));
#12329=CARTESIAN_POINT('Ctrl Pts',(-0.0158075115832676,-0.325,0.4));
#12330=CARTESIAN_POINT('Ctrl Pts',(-0.0325978607437828,-0.328180693480621,
0.398970551469948));
#12331=CARTESIAN_POINT('Ctrl Pts',(-0.0633657881355918,-0.340970918840894,
0.395252954914593));
#12332=CARTESIAN_POINT('Ctrl Pts',(-0.0773514949786257,-0.350574799681989,
0.392612801026882));
#12333=CARTESIAN_POINT('Ctrl Pts',(-0.0994291026068839,-0.372652407310247,
0.38761064154154));
#12334=CARTESIAN_POINT('Ctrl Pts',(-0.109029967924066,-0.38663653976279,
0.384911758361269));
#12335=CARTESIAN_POINT('Ctrl Pts',(-0.121817958968287,-0.41739870290668,
0.381057715344782));
#12336=CARTESIAN_POINT('Ctrl Pts',(-0.125,-0.434186899370797,0.379967103839267));
#12337=CARTESIAN_POINT('Ctrl Pts',(-0.125,-0.45,0.379967103839267));
#12338=CARTESIAN_POINT('Ctrl Pts',(-0.125,-0.45,0.379967103839267));
#12339=CARTESIAN_POINT('Ctrl Pts',(-0.125,-0.465813100629203,0.379967103839267));
#12340=CARTESIAN_POINT('Ctrl Pts',(-0.121817958968287,-0.48260129709332,
0.381057715344782));
#12341=CARTESIAN_POINT('Ctrl Pts',(-0.109029967924066,-0.51336346023721,
0.384911758361269));
#12342=CARTESIAN_POINT('Ctrl Pts',(-0.0994291026068839,-0.527347592689753,
0.38761064154154));
#12343=CARTESIAN_POINT('Ctrl Pts',(-0.0773514949786256,-0.549425200318011,
0.392612801026882));
#12344=CARTESIAN_POINT('Ctrl Pts',(-0.0633657881355917,-0.559029081159106,
0.395252954914593));
#12345=CARTESIAN_POINT('Ctrl Pts',(-0.0325978607437828,-0.571819306519379,
0.398970551469948));
#12346=CARTESIAN_POINT('Ctrl Pts',(-0.0158075115832675,-0.575,0.4));
#12347=CARTESIAN_POINT('Ctrl Pts',(0.0158075115832676,-0.575,0.4));
#12348=CARTESIAN_POINT('Ctrl Pts',(0.0325978607437828,-0.571819306519379,
0.398970551469948));
#12349=CARTESIAN_POINT('Ctrl Pts',(0.0633657881355917,-0.559029081159106,
0.395252954914593));
#12350=CARTESIAN_POINT('Ctrl Pts',(0.0773514949786257,-0.549425200318011,
0.392612801026882));
#12351=CARTESIAN_POINT('Ctrl Pts',(0.0994291026068839,-0.527347592689753,
0.38761064154154));
#12352=CARTESIAN_POINT('Ctrl Pts',(0.109029967924066,-0.51336346023721,
0.384911758361269));
#12353=CARTESIAN_POINT('Ctrl Pts',(0.121817958968287,-0.48260129709332,
0.381057715344782));
#12354=CARTESIAN_POINT('Ctrl Pts',(0.125,-0.465813100629203,0.379967103839267));
#12355=CARTESIAN_POINT('Ctrl Pts',(0.125,-0.45,0.379967103839267));
#12356=CARTESIAN_POINT('',(-0.125,-0.45,0.));
#12357=CARTESIAN_POINT('Origin',(0.,0.,0.));
#12358=CARTESIAN_POINT('',(-0.4,-0.8,4.89858719658941E-17));
#12359=CARTESIAN_POINT('Origin',(0.,-0.8,0.));
#12360=CARTESIAN_POINT('',(-0.4,0.,4.89858719658941E-17));
#12361=CARTESIAN_POINT('',(-0.4,0.85,-4.89858719658941E-17));
#12362=CARTESIAN_POINT('',(-0.4,0.,4.89858719658941E-17));
#12363=CARTESIAN_POINT('Origin',(0.,0.85,0.));
#12364=CARTESIAN_POINT('Origin',(0.,-0.8,0.));
#12365=CARTESIAN_POINT('Origin',(0.,0.,0.));
#12366=CARTESIAN_POINT('',(-0.8,0.,9.79717439317883E-17));
#12367=CARTESIAN_POINT('Origin',(0.,0.,0.));
#12368=CARTESIAN_POINT('',(0.595438916863769,0.,0.137993139022126));
#12369=CARTESIAN_POINT('',(0.562830534889751,0.,0.238351419397483));
#12370=CARTESIAN_POINT('Origin',(0.562758945330873,0.,0.182851465569258));
#12371=CARTESIAN_POINT('',(0.523653836874034,0.,0.315240018494132));
#12372=CARTESIAN_POINT('Origin',(0.,0.,0.));
#12373=CARTESIAN_POINT('',(0.461629008549572,0.,0.40060987082025));
#12374=CARTESIAN_POINT('Origin',(0.478711351753049,0.,0.347804155687524));
#12375=CARTESIAN_POINT('',(0.40060987082025,0.,0.461629008549572));
#12376=CARTESIAN_POINT('Origin',(0.,0.,0.));
#12377=CARTESIAN_POINT('',(0.315240018494132,0.,0.523653836874034));
#12378=CARTESIAN_POINT('Origin',(0.347804155687523,0.,0.478711351753049));
#12379=CARTESIAN_POINT('',(0.238351419397483,0.,0.562830534889751));
#12380=CARTESIAN_POINT('Origin',(0.,0.,0.));
#12381=CARTESIAN_POINT('',(0.137993139022126,0.,0.595438916863769));
#12382=CARTESIAN_POINT('Origin',(0.182851465569258,0.,0.562758945330873));
#12383=CARTESIAN_POINT('',(0.0527614703521001,0.,0.608938287003997));
#12384=CARTESIAN_POINT('Origin',(0.,0.,0.));
#12385=CARTESIAN_POINT('',(-0.0527614703521003,0.,0.608938287003997));
#12386=CARTESIAN_POINT('Origin',(-1.08697158783324E-16,0.,0.591719772367581));
#12387=CARTESIAN_POINT('',(-0.137993139022126,0.,0.595438916863769));
#12388=CARTESIAN_POINT('Origin',(0.,0.,0.));
#12389=CARTESIAN_POINT('',(-0.238351419397483,0.,0.562830534889751));
#12390=CARTESIAN_POINT('Origin',(-0.182851465569258,0.,0.562758945330873));
#12391=CARTESIAN_POINT('',(-0.315240018494132,0.,0.523653836874034));
#12392=CARTESIAN_POINT('Origin',(0.,0.,0.));
#12393=CARTESIAN_POINT('',(-0.40060987082025,0.,0.461629008549572));
#12394=CARTESIAN_POINT('Origin',(-0.347804155687524,0.,0.478711351753049));
#12395=CARTESIAN_POINT('',(-0.461629008549572,0.,0.40060987082025));
#12396=CARTESIAN_POINT('Origin',(0.,0.,0.));
#12397=CARTESIAN_POINT('',(-0.523653836874034,0.,0.315240018494132));
#12398=CARTESIAN_POINT('Origin',(-0.478711351753049,0.,0.347804155687524));
#12399=CARTESIAN_POINT('',(-0.562830534889751,0.,0.238351419397483));
#12400=CARTESIAN_POINT('Origin',(0.,0.,0.));
#12401=CARTESIAN_POINT('',(-0.595438916863769,0.,0.137993139022126));
#12402=CARTESIAN_POINT('Origin',(-0.562758945330873,0.,0.182851465569258));
#12403=CARTESIAN_POINT('',(-0.608938287003997,0.,0.0527614703521002));
#12404=CARTESIAN_POINT('Origin',(0.,0.,0.));
#12405=CARTESIAN_POINT('',(-0.608938287003997,0.,-0.0527614703521003));
#12406=CARTESIAN_POINT('Origin',(-0.591719772367581,0.,-7.24647725222159E-17));
#12407=CARTESIAN_POINT('',(-0.595438916863769,0.,-0.137993139022126));
#12408=CARTESIAN_POINT('Origin',(0.,0.,0.));
#12409=CARTESIAN_POINT('',(-0.562830534889751,0.,-0.238351419397483));
#12410=CARTESIAN_POINT('Origin',(-0.562758945330873,0.,-0.182851465569258));
#12411=CARTESIAN_POINT('',(-0.523653836874034,0.,-0.315240018494132));
#12412=CARTESIAN_POINT('Origin',(0.,0.,0.));
#12413=CARTESIAN_POINT('',(-0.461629008549572,0.,-0.40060987082025));
#12414=CARTESIAN_POINT('Origin',(-0.478711351753049,0.,-0.347804155687524));
#12415=CARTESIAN_POINT('',(-0.40060987082025,0.,-0.461629008549572));
#12416=CARTESIAN_POINT('Origin',(0.,0.,0.));
#12417=CARTESIAN_POINT('',(-0.315240018494132,0.,-0.523653836874034));
#12418=CARTESIAN_POINT('Origin',(-0.347804155687524,0.,-0.478711351753049));
#12419=CARTESIAN_POINT('',(-0.238351419397483,0.,-0.562830534889751));
#12420=CARTESIAN_POINT('Origin',(0.,0.,0.));
#12421=CARTESIAN_POINT('',(-0.137993139022126,0.,-0.595438916863769));
#12422=CARTESIAN_POINT('Origin',(-0.182851465569258,0.,-0.562758945330873));
#12423=CARTESIAN_POINT('',(-0.0527614703521002,0.,-0.608938287003997));
#12424=CARTESIAN_POINT('Origin',(0.,0.,0.));
#12425=CARTESIAN_POINT('',(0.0527614703521003,0.,-0.608938287003997));
#12426=CARTESIAN_POINT('Origin',(3.6232386261108E-17,0.,-0.591719772367581));
#12427=CARTESIAN_POINT('',(0.137993139022126,0.,-0.595438916863769));
#12428=CARTESIAN_POINT('Origin',(0.,0.,0.));
#12429=CARTESIAN_POINT('',(0.238351419397483,0.,-0.562830534889751));
#12430=CARTESIAN_POINT('Origin',(0.182851465569258,0.,-0.562758945330873));
#12431=CARTESIAN_POINT('',(0.315240018494132,0.,-0.523653836874034));
#12432=CARTESIAN_POINT('Origin',(0.,0.,0.));
#12433=CARTESIAN_POINT('',(0.40060987082025,0.,-0.461629008549572));
#12434=CARTESIAN_POINT('Origin',(0.347804155687524,0.,-0.478711351753049));
#12435=CARTESIAN_POINT('',(0.461629008549572,0.,-0.40060987082025));
#12436=CARTESIAN_POINT('Origin',(0.,0.,0.));
#12437=CARTESIAN_POINT('',(0.523653836874034,0.,-0.315240018494132));
#12438=CARTESIAN_POINT('Origin',(0.478711351753049,0.,-0.347804155687524));
#12439=CARTESIAN_POINT('',(0.562830534889751,0.,-0.238351419397483));
#12440=CARTESIAN_POINT('Origin',(0.,0.,0.));
#12441=CARTESIAN_POINT('',(0.595438916863769,0.,-0.137993139022126));
#12442=CARTESIAN_POINT('Origin',(0.562758945330873,0.,-0.182851465569258));
#12443=CARTESIAN_POINT('',(0.608938287003997,0.,-0.0527614703521001));
#12444=CARTESIAN_POINT('Origin',(0.,0.,0.));
#12445=CARTESIAN_POINT('',(0.608938287003997,0.,0.0527614703521001));
#12446=CARTESIAN_POINT('Origin',(0.591719772367581,0.,0.));
#12447=CARTESIAN_POINT('Origin',(0.,0.,0.));
#12448=CARTESIAN_POINT('Origin',(0.,0.,0.));
#12449=CARTESIAN_POINT('',(-0.8,-0.1,9.79717439317883E-17));
#12450=CARTESIAN_POINT('Origin',(0.,-0.1,0.));
#12451=CARTESIAN_POINT('',(-0.8,0.,-9.79717439317883E-17));
#12452=CARTESIAN_POINT('Origin',(0.,-0.1,0.));
#12453=CARTESIAN_POINT('Origin',(0.,0.75,0.));
#12454=CARTESIAN_POINT('',(-0.8,0.75,9.79717439317883E-17));
#12455=CARTESIAN_POINT('Origin',(0.,0.75,0.));
#12456=CARTESIAN_POINT('',(0.562830534889751,0.75,0.238351419397483));
#12457=CARTESIAN_POINT('',(0.595438916863769,0.75,0.137993139022126));
#12458=CARTESIAN_POINT('Origin',(0.562758945330873,0.75,0.182851465569258));
#12459=CARTESIAN_POINT('',(0.608938287003997,0.75,0.0527614703521002));
#12460=CARTESIAN_POINT('Origin',(0.,0.75,0.));
#12461=CARTESIAN_POINT('',(0.608938287003997,0.75,-0.0527614703521002));
#12462=CARTESIAN_POINT('Origin',(0.591719772367581,0.75,0.));
#12463=CARTESIAN_POINT('',(0.595438916863769,0.75,-0.137993139022126));
#12464=CARTESIAN_POINT('Origin',(0.,0.75,0.));
#12465=CARTESIAN_POINT('',(0.562830534889751,0.75,-0.238351419397483));
#12466=CARTESIAN_POINT('Origin',(0.562758945330873,0.75,-0.182851465569258));
#12467=CARTESIAN_POINT('',(0.523653836874034,0.75,-0.315240018494132));
#12468=CARTESIAN_POINT('Origin',(0.,0.75,0.));
#12469=CARTESIAN_POINT('',(0.461629008549572,0.75,-0.40060987082025));
#12470=CARTESIAN_POINT('Origin',(0.478711351753049,0.75,-0.347804155687524));
#12471=CARTESIAN_POINT('',(0.40060987082025,0.75,-0.461629008549572));
#12472=CARTESIAN_POINT('Origin',(0.,0.75,0.));
#12473=CARTESIAN_POINT('',(0.315240018494132,0.75,-0.523653836874034));
#12474=CARTESIAN_POINT('Origin',(0.347804155687524,0.75,-0.478711351753049));
#12475=CARTESIAN_POINT('',(0.238351419397483,0.75,-0.562830534889751));
#12476=CARTESIAN_POINT('Origin',(0.,0.75,0.));
#12477=CARTESIAN_POINT('',(0.137993139022126,0.75,-0.595438916863769));
#12478=CARTESIAN_POINT('Origin',(0.182851465569258,0.75,-0.562758945330873));
#12479=CARTESIAN_POINT('',(0.0527614703521003,0.75,-0.608938287003997));
#12480=CARTESIAN_POINT('Origin',(0.,0.75,0.));
#12481=CARTESIAN_POINT('',(-0.0527614703521002,0.75,-0.608938287003997));
#12482=CARTESIAN_POINT('Origin',(3.6232386261108E-17,0.75,-0.591719772367581));
#12483=CARTESIAN_POINT('',(-0.137993139022126,0.75,-0.595438916863769));
#12484=CARTESIAN_POINT('Origin',(0.,0.75,0.));
#12485=CARTESIAN_POINT('',(-0.238351419397483,0.75,-0.562830534889751));
#12486=CARTESIAN_POINT('Origin',(-0.182851465569258,0.75,-0.562758945330873));
#12487=CARTESIAN_POINT('',(-0.315240018494132,0.75,-0.523653836874034));
#12488=CARTESIAN_POINT('Origin',(0.,0.75,0.));
#12489=CARTESIAN_POINT('',(-0.40060987082025,0.75,-0.461629008549572));
#12490=CARTESIAN_POINT('Origin',(-0.347804155687524,0.75,-0.478711351753049));
#12491=CARTESIAN_POINT('',(-0.461629008549572,0.75,-0.40060987082025));
#12492=CARTESIAN_POINT('Origin',(0.,0.75,0.));
#12493=CARTESIAN_POINT('',(-0.523653836874034,0.75,-0.315240018494132));
#12494=CARTESIAN_POINT('Origin',(-0.478711351753049,0.75,-0.347804155687524));
#12495=CARTESIAN_POINT('',(-0.562830534889751,0.75,-0.238351419397483));
#12496=CARTESIAN_POINT('Origin',(0.,0.75,0.));
#12497=CARTESIAN_POINT('',(-0.595438916863769,0.75,-0.137993139022126));
#12498=CARTESIAN_POINT('Origin',(-0.562758945330873,0.75,-0.182851465569258));
#12499=CARTESIAN_POINT('',(-0.608938287003997,0.75,-0.0527614703521003));
#12500=CARTESIAN_POINT('Origin',(0.,0.75,0.));
#12501=CARTESIAN_POINT('',(-0.608938287003997,0.75,0.0527614703521002));
#12502=CARTESIAN_POINT('Origin',(-0.591719772367581,0.75,-7.24647725222159E-17));
#12503=CARTESIAN_POINT('',(-0.595438916863769,0.75,0.137993139022126));
#12504=CARTESIAN_POINT('Origin',(0.,0.75,0.));
#12505=CARTESIAN_POINT('',(-0.562830534889751,0.75,0.238351419397483));
#12506=CARTESIAN_POINT('Origin',(-0.562758945330873,0.75,0.182851465569258));
#12507=CARTESIAN_POINT('',(-0.523653836874034,0.75,0.315240018494132));
#12508=CARTESIAN_POINT('Origin',(0.,0.75,0.));
#12509=CARTESIAN_POINT('',(-0.461629008549572,0.75,0.40060987082025));
#12510=CARTESIAN_POINT('Origin',(-0.478711351753049,0.75,0.347804155687524));
#12511=CARTESIAN_POINT('',(-0.40060987082025,0.75,0.461629008549572));
#12512=CARTESIAN_POINT('Origin',(0.,0.75,0.));
#12513=CARTESIAN_POINT('',(-0.315240018494132,0.75,0.523653836874034));
#12514=CARTESIAN_POINT('Origin',(-0.347804155687524,0.75,0.478711351753049));
#12515=CARTESIAN_POINT('',(-0.238351419397483,0.75,0.562830534889751));
#12516=CARTESIAN_POINT('Origin',(0.,0.75,0.));
#12517=CARTESIAN_POINT('',(-0.137993139022126,0.75,0.595438916863769));
#12518=CARTESIAN_POINT('Origin',(-0.182851465569258,0.75,0.562758945330873));
#12519=CARTESIAN_POINT('',(-0.0527614703521003,0.75,0.608938287003997));
#12520=CARTESIAN_POINT('Origin',(0.,0.75,0.));
#12521=CARTESIAN_POINT('',(0.0527614703521001,0.75,0.608938287003997));
#12522=CARTESIAN_POINT('Origin',(-1.08697158783324E-16,0.75,0.591719772367581));
#12523=CARTESIAN_POINT('',(0.137993139022126,0.75,0.595438916863769));
#12524=CARTESIAN_POINT('Origin',(0.,0.75,0.));
#12525=CARTESIAN_POINT('',(0.238351419397483,0.75,0.562830534889751));
#12526=CARTESIAN_POINT('Origin',(0.182851465569258,0.75,0.562758945330873));
#12527=CARTESIAN_POINT('',(0.315240018494132,0.75,0.523653836874034));
#12528=CARTESIAN_POINT('Origin',(0.,0.75,0.));
#12529=CARTESIAN_POINT('',(0.40060987082025,0.75,0.461629008549572));
#12530=CARTESIAN_POINT('Origin',(0.347804155687523,0.75,0.478711351753049));
#12531=CARTESIAN_POINT('',(0.461629008549572,0.75,0.40060987082025));
#12532=CARTESIAN_POINT('Origin',(0.,0.75,0.));
#12533=CARTESIAN_POINT('',(0.523653836874034,0.75,0.315240018494132));
#12534=CARTESIAN_POINT('Origin',(0.478711351753049,0.75,0.347804155687524));
#12535=CARTESIAN_POINT('Origin',(0.,0.75,0.));
#12536=CARTESIAN_POINT('Origin',(0.,0.75,0.));
#12537=CARTESIAN_POINT('',(-0.8,0.85,9.79717439317883E-17));
#12538=CARTESIAN_POINT('Origin',(0.,0.85,0.));
#12539=CARTESIAN_POINT('',(-0.8,0.75,9.79717439317883E-17));
#12540=CARTESIAN_POINT('Origin',(0.,0.85,0.));
#12541=CARTESIAN_POINT('Origin',(0.562758945330873,0.,0.182851465569258));
#12542=CARTESIAN_POINT('',(0.595438916863769,0.,0.137993139022126));
#12543=CARTESIAN_POINT('',(0.562830534889751,0.,0.238351419397483));
#12544=CARTESIAN_POINT('Origin',(0.,0.,0.));
#12545=CARTESIAN_POINT('',(0.523653836874034,0.,0.315240018494132));
#12546=CARTESIAN_POINT('Origin',(0.478711351753049,0.,0.347804155687524));
#12547=CARTESIAN_POINT('',(0.461629008549572,0.,0.40060987082025));
#12548=CARTESIAN_POINT('Origin',(0.,0.,0.));
#12549=CARTESIAN_POINT('',(0.40060987082025,0.,0.461629008549572));
#12550=CARTESIAN_POINT('Origin',(0.347804155687523,0.,0.478711351753049));
#12551=CARTESIAN_POINT('',(0.315240018494132,0.,0.523653836874034));
#12552=CARTESIAN_POINT('Origin',(0.,0.,0.));
#12553=CARTESIAN_POINT('',(0.238351419397483,0.,0.562830534889751));
#12554=CARTESIAN_POINT('Origin',(0.182851465569258,0.,0.562758945330873));
#12555=CARTESIAN_POINT('',(0.137993139022126,0.,0.595438916863769));
#12556=CARTESIAN_POINT('Origin',(0.,0.,0.));
#12557=CARTESIAN_POINT('',(0.0527614703521,0.,0.608938287003997));
#12558=CARTESIAN_POINT('Origin',(-1.08697158783324E-16,0.,0.591719772367581));
#12559=CARTESIAN_POINT('',(-0.0527614703521002,0.,0.608938287003997));
#12560=CARTESIAN_POINT('Origin',(0.,0.,0.));
#12561=CARTESIAN_POINT('',(-0.137993139022126,0.,0.595438916863769));
#12562=CARTESIAN_POINT('Origin',(-0.182851465569258,0.,0.562758945330873));
#12563=CARTESIAN_POINT('',(-0.238351419397483,0.,0.562830534889751));
#12564=CARTESIAN_POINT('Origin',(0.,0.,0.));
#12565=CARTESIAN_POINT('',(-0.315240018494132,0.,0.523653836874034));
#12566=CARTESIAN_POINT('Origin',(-0.347804155687524,0.,0.478711351753049));
#12567=CARTESIAN_POINT('',(-0.40060987082025,0.,0.461629008549572));
#12568=CARTESIAN_POINT('Origin',(0.,0.,0.));
#12569=CARTESIAN_POINT('',(-0.461629008549572,0.,0.40060987082025));
#12570=CARTESIAN_POINT('Origin',(-0.478711351753049,0.,0.347804155687524));
#12571=CARTESIAN_POINT('',(-0.523653836874034,0.,0.315240018494132));
#12572=CARTESIAN_POINT('Origin',(0.,0.,0.));
#12573=CARTESIAN_POINT('',(-0.562830534889751,0.,0.238351419397483));
#12574=CARTESIAN_POINT('Origin',(-0.562758945330873,0.,0.182851465569258));
#12575=CARTESIAN_POINT('',(-0.595438916863769,0.,0.137993139022126));
#12576=CARTESIAN_POINT('Origin',(0.,0.,0.));
#12577=CARTESIAN_POINT('',(-0.608938287003997,0.,0.0527614703521));
#12578=CARTESIAN_POINT('Origin',(-0.591719772367581,0.,-7.24647725222159E-17));
#12579=CARTESIAN_POINT('',(-0.608938287003997,0.,-0.0527614703521002));
#12580=CARTESIAN_POINT('Origin',(0.,0.,0.));
#12581=CARTESIAN_POINT('',(-0.595438916863769,0.,-0.137993139022126));
#12582=CARTESIAN_POINT('Origin',(-0.562758945330873,0.,-0.182851465569258));
#12583=CARTESIAN_POINT('',(-0.562830534889751,0.,-0.238351419397483));
#12584=CARTESIAN_POINT('Origin',(0.,0.,0.));
#12585=CARTESIAN_POINT('',(-0.523653836874034,0.,-0.315240018494132));
#12586=CARTESIAN_POINT('Origin',(-0.478711351753049,0.,-0.347804155687524));
#12587=CARTESIAN_POINT('',(-0.461629008549572,0.,-0.40060987082025));
#12588=CARTESIAN_POINT('Origin',(0.,0.,0.));
#12589=CARTESIAN_POINT('',(-0.40060987082025,0.,-0.461629008549572));
#12590=CARTESIAN_POINT('Origin',(-0.347804155687524,0.,-0.478711351753049));
#12591=CARTESIAN_POINT('',(-0.315240018494132,0.,-0.523653836874034));
#12592=CARTESIAN_POINT('Origin',(0.,0.,0.));
#12593=CARTESIAN_POINT('',(-0.238351419397483,0.,-0.562830534889751));
#12594=CARTESIAN_POINT('Origin',(-0.182851465569258,0.,-0.562758945330873));
#12595=CARTESIAN_POINT('',(-0.137993139022126,0.,-0.595438916863769));
#12596=CARTESIAN_POINT('Origin',(0.,0.,0.));
#12597=CARTESIAN_POINT('',(-0.0527614703521,0.,-0.608938287003997));
#12598=CARTESIAN_POINT('Origin',(3.6232386261108E-17,0.,-0.591719772367581));
#12599=CARTESIAN_POINT('',(0.0527614703521001,0.,-0.608938287003997));
#12600=CARTESIAN_POINT('Origin',(0.,0.,0.));
#12601=CARTESIAN_POINT('',(0.137993139022126,0.,-0.595438916863769));
#12602=CARTESIAN_POINT('Origin',(0.182851465569258,0.,-0.562758945330873));
#12603=CARTESIAN_POINT('',(0.238351419397483,0.,-0.562830534889751));
#12604=CARTESIAN_POINT('Origin',(0.,0.,0.));
#12605=CARTESIAN_POINT('',(0.315240018494132,0.,-0.523653836874034));
#12606=CARTESIAN_POINT('Origin',(0.347804155687524,0.,-0.478711351753049));
#12607=CARTESIAN_POINT('',(0.40060987082025,0.,-0.461629008549572));
#12608=CARTESIAN_POINT('Origin',(0.,0.,0.));
#12609=CARTESIAN_POINT('',(0.461629008549572,0.,-0.40060987082025));
#12610=CARTESIAN_POINT('Origin',(0.478711351753049,0.,-0.347804155687524));
#12611=CARTESIAN_POINT('',(0.523653836874034,0.,-0.315240018494132));
#12612=CARTESIAN_POINT('Origin',(0.,0.,0.));
#12613=CARTESIAN_POINT('',(0.562830534889751,0.,-0.238351419397483));
#12614=CARTESIAN_POINT('Origin',(0.562758945330873,0.,-0.182851465569258));
#12615=CARTESIAN_POINT('',(0.595438916863769,0.,-0.137993139022126));
#12616=CARTESIAN_POINT('Origin',(0.,0.,0.));
#12617=CARTESIAN_POINT('',(0.608938287003997,0.,0.0527614703521001));
#12618=CARTESIAN_POINT('Origin',(0.591719772367581,0.,0.));
#12619=CARTESIAN_POINT('',(0.608938287003997,0.,-0.0527614703521001));
#12620=CARTESIAN_POINT('Origin',(0.,0.,0.));
#12737=UNCERTAINTY_MEASURE_WITH_UNIT(LENGTH_MEASURE(0.001),#12780,
'DISTANCE_ACCURACY_VALUE',
'Maximum model space distance between geometric entities at asserted c
onnectivities');
#12739=UNCERTAINTY_MEASURE_WITH_UNIT(LENGTH_MEASURE(0.001),#12780,
'DISTANCE_ACCURACY_VALUE',
'Maximum model space distance between geometric entities at asserted c
onnectivities');
#12777=(
GEOMETRIC_REPRESENTATION_CONTEXT(3)
GLOBAL_UNCERTAINTY_ASSIGNED_CONTEXT((#12737))
GLOBAL_UNIT_ASSIGNED_CONTEXT((#12780,#12782,#12783))
REPRESENTATION_CONTEXT('','3D')
);
#12779=(
GEOMETRIC_REPRESENTATION_CONTEXT(3)
GLOBAL_UNCERTAINTY_ASSIGNED_CONTEXT((#12739))
GLOBAL_UNIT_ASSIGNED_CONTEXT((#12780,#12782,#12783))
REPRESENTATION_CONTEXT('','3D')
);
#12780=(
LENGTH_UNIT()
NAMED_UNIT(*)
SI_UNIT(.CENTI.,.METRE.)
);
#12782=(
NAMED_UNIT(*)
PLANE_ANGLE_UNIT()
SI_UNIT($,.RADIAN.)
);
#12783=(
NAMED_UNIT(*)
SI_UNIT($,.STERADIAN.)
SOLID_ANGLE_UNIT()
);
#12821=SHAPE_DEFINITION_REPRESENTATION(#12908,#12960);
#12908=PRODUCT_DEFINITION_SHAPE('',$,#13000);
#12960=SHAPE_REPRESENTATION('',(#7254),#12777);
#12962=PRODUCT_DEFINITION_CONTEXT('part definition',#13081,'design');
#13000=PRODUCT_DEFINITION(
'Timing Pulley - 2 mm Pitch, 20 Teeth, 8 mm Bore',
'Timing Pulley - 2 mm Pitch, 20 Teeth, 8 mm Bore',#13039,#12962);
#13039=PRODUCT_DEFINITION_FORMATION('',$,#13120);
#13081=APPLICATION_CONTEXT(
'Core Data for Automotive Mechanical Design Process');
#13082=PRODUCT_CONTEXT('part definition',#13081,'mechanical');
#13120=PRODUCT('Timing Pulley - 2 mm Pitch, 20 Teeth, 8 mm Bore',
'Timing Pulley - 2 mm Pitch, 20 Teeth, 8 mm Bore',
'Timing Pulley - 2 mm Pitch, 20 Teeth, 8 mm Bore',(#13082));
#13192=COLOUR_RGB('Off White',0.89,0.88,0.83);
#13193=FILL_AREA_STYLE_COLOUR('',#13192);
#13194=FILL_AREA_STYLE('',(#13193));
#13195=SURFACE_STYLE_FILL_AREA(#13194);
#13196=SURFACE_SIDE_STYLE('',(#13195));
#13197=SURFACE_STYLE_USAGE(.BOTH.,#13196);
#13198=PRESENTATION_STYLE_ASSIGNMENT((#13197));
ENDSEC;
END-ISO-10303-21;
